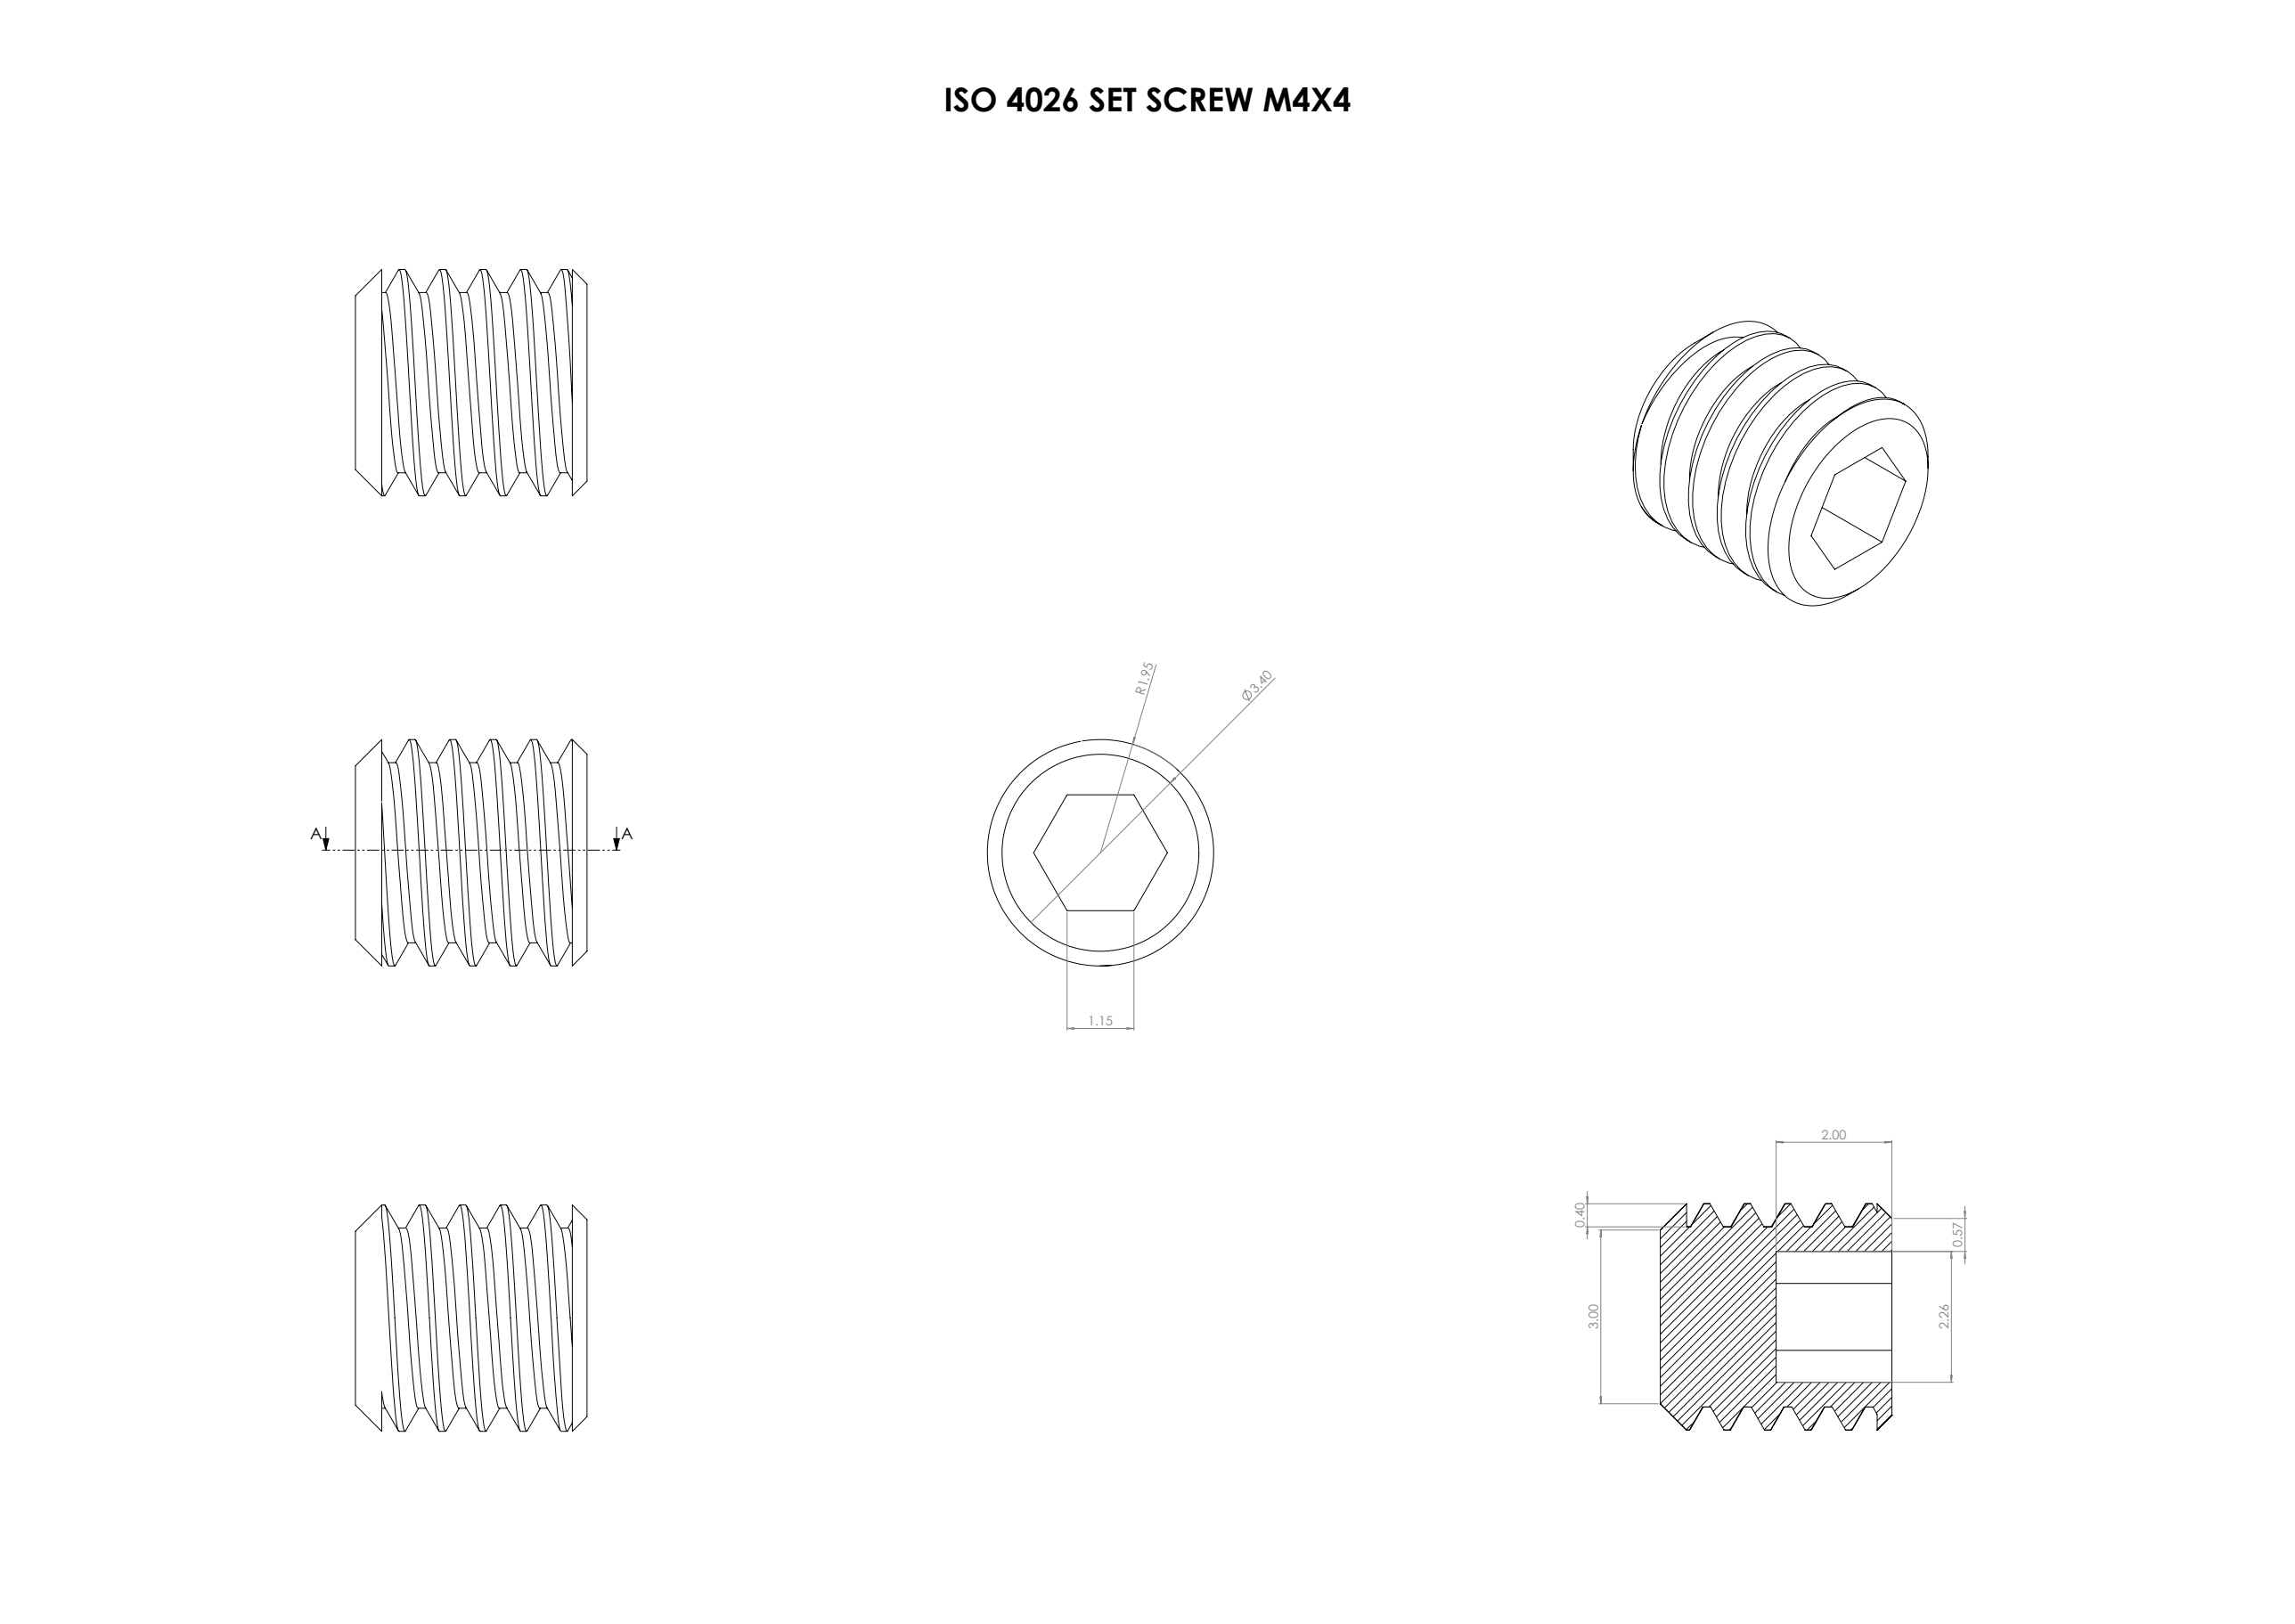
ISO-10303-21;
HEADER;
/* Generated by software containing ST-Developer
 * from STEP Tools, Inc. (www.steptools.com) 
 */

FILE_DESCRIPTION(
/* description */ (''),
/* implementation_level */ '2;1');

FILE_NAME(
/* name */ '10_ISO_4026_Set_Screw_M4x4.step',
/* time_stamp */ '2026-10-21T01:59:45-07:00',
/* author */ (''),
/* organization */ (''),
/* preprocessor_version */ 'ST-DEVELOPER v20.2',
/* originating_system */ 'Autodesk Translation Framework v15.15.0.0',
/* authorisation */ '');

FILE_SCHEMA (('AUTOMOTIVE_DESIGN { 1 0 10303 214 3 1 1 }'));
ENDSEC;

DATA;
#10=MECHANICAL_DESIGN_GEOMETRIC_PRESENTATION_REPRESENTATION('',(#478),#18281);
#184=B_SPLINE_SURFACE_WITH_KNOTS('',3,3,((#15681,#15682,#15683,#15684,#15685,
#15686,#15687,#15688,#15689,#15690,#15691,#15692,#15693,#15694,#15695,#15696,
#15697,#15698,#15699,#15700,#15701,#15702,#15703,#15704,#15705,#15706,#15707,
#15708,#15709,#15710,#15711,#15712,#15713,#15714,#15715),(#15716,#15717,
#15718,#15719,#15720,#15721,#15722,#15723,#15724,#15725,#15726,#15727,#15728,
#15729,#15730,#15731,#15732,#15733,#15734,#15735,#15736,#15737,#15738,#15739,
#15740,#15741,#15742,#15743,#15744,#15745,#15746,#15747,#15748,#15749,#15750),
(#15751,#15752,#15753,#15754,#15755,#15756,#15757,#15758,#15759,#15760,
#15761,#15762,#15763,#15764,#15765,#15766,#15767,#15768,#15769,#15770,#15771,
#15772,#15773,#15774,#15775,#15776,#15777,#15778,#15779,#15780,#15781,#15782,
#15783,#15784,#15785),(#15786,#15787,#15788,#15789,#15790,#15791,#15792,
#15793,#15794,#15795,#15796,#15797,#15798,#15799,#15800,#15801,#15802,#15803,
#15804,#15805,#15806,#15807,#15808,#15809,#15810,#15811,#15812,#15813,#15814,
#15815,#15816,#15817,#15818,#15819,#15820)),.UNSPECIFIED.,.F.,.F.,.F.,(4,
4),(4,1,1,1,1,1,1,1,1,1,1,1,1,1,1,1,1,1,1,1,1,1,1,1,1,1,1,1,1,1,1,1,4),
(0.,0.0460148164544132),(8.31058692273978,9.29852639258487,10.28646586243,
11.274405332275,12.2623448021201,13.2502842719652,14.2382237418103,15.2261632116554,
16.2141026815005,17.2020421513455,18.1899816211906,19.1779210910357,20.1658605608808,
21.1538000307259,22.141739500571,23.129678970416,24.1176184402611,25.1055579101062,
26.0934973799513,27.0814368497964,28.0693763196415,29.0573157894865,30.0452552593316,
31.0331947291767,32.0211341990218,33.0090736688669,33.997013138712,34.9849526085571,
35.9728920784021,36.9608315482472,37.9487710180923,38.9367104879374,39.9246499577825),
 .UNSPECIFIED.);
#185=B_SPLINE_SURFACE_WITH_KNOTS('',3,3,((#16035,#16036,#16037,#16038,#16039,
#16040,#16041,#16042,#16043,#16044,#16045,#16046,#16047,#16048,#16049,#16050,
#16051,#16052,#16053,#16054,#16055,#16056,#16057,#16058,#16059,#16060,#16061,
#16062,#16063,#16064,#16065,#16066,#16067,#16068,#16069),(#16070,#16071,
#16072,#16073,#16074,#16075,#16076,#16077,#16078,#16079,#16080,#16081,#16082,
#16083,#16084,#16085,#16086,#16087,#16088,#16089,#16090,#16091,#16092,#16093,
#16094,#16095,#16096,#16097,#16098,#16099,#16100,#16101,#16102,#16103,#16104),
(#16105,#16106,#16107,#16108,#16109,#16110,#16111,#16112,#16113,#16114,
#16115,#16116,#16117,#16118,#16119,#16120,#16121,#16122,#16123,#16124,#16125,
#16126,#16127,#16128,#16129,#16130,#16131,#16132,#16133,#16134,#16135,#16136,
#16137,#16138,#16139),(#16140,#16141,#16142,#16143,#16144,#16145,#16146,
#16147,#16148,#16149,#16150,#16151,#16152,#16153,#16154,#16155,#16156,#16157,
#16158,#16159,#16160,#16161,#16162,#16163,#16164,#16165,#16166,#16167,#16168,
#16169,#16170,#16171,#16172,#16173,#16174)),.UNSPECIFIED.,.F.,.F.,.F.,(4,
4),(4,1,1,1,1,1,1,1,1,1,1,1,1,1,1,1,1,1,1,1,1,1,1,1,1,1,1,1,1,1,1,1,4),
(0.,0.0460148164544132),(11.6154215191107,12.6033609889557,13.5913004588008,
14.5792399286459,15.567179398491,16.5551188683361,17.5430583381812,18.5309978080262,
19.5189372778713,20.5068767477164,21.4948162175615,22.4827556874066,23.4706951572517,
24.4586346270967,25.4465740969418,26.4345135667869,27.422453036632,28.4103925064771,
29.3983319763222,30.3862714461672,31.3742109160123,32.3621503858574,33.3500898557025,
34.3380293255476,35.3259687953927,36.3139082652377,37.3018477350828,38.2897872049279,
39.277726674773,40.2656661446181,41.2536056144632,42.2415450843083,43.2294845541533),
 .UNSPECIFIED.);
#285=B_SPLINE_CURVE_WITH_KNOTS('',3,(#15173,#15174,#15175,#15176,#15177,
#15178,#15179,#15180,#15181,#15182),.UNSPECIFIED.,.F.,.F.,(4,3,3,4),(-4.09254174883831,
-3.95175787938034,-2.96381840953525,-2.0651401332781),.UNSPECIFIED.);
#286=B_SPLINE_CURVE_WITH_KNOTS('',3,(#15185,#15186,#15187,#15188,#15189,
#15190,#15191),.UNSPECIFIED.,.F.,.F.,(4,3,4),(0.,0.987939469845084,1.11419103802959),
 .UNSPECIFIED.);
#287=B_SPLINE_CURVE_WITH_KNOTS('',3,(#15196,#15197,#15198,#15199,#15200,
#15201,#15202,#15203,#15204,#15205,#15206,#15207,#15208,#15209,#15210,#15211,
#15212,#15213,#15214,#15215,#15216,#15217),.UNSPECIFIED.,.F.,.F.,(4,3,3,
3,3,3,3,4),(-10.3757270560179,-9.87939469845084,-8.89145522860576,-7.90351575876067,
-6.91557628891559,-5.92763681907051,-4.93969734922542,-4.09254174883831),
 .UNSPECIFIED.);
#288=B_SPLINE_CURVE_WITH_KNOTS('',3,(#15218,#15219,#15220,#15221,#15222,
#15223,#15224,#15225,#15226,#15227,#15228,#15229,#15230,#15231,#15232,#15233,
#15234,#15235,#15236,#15237,#15238,#15239),.UNSPECIFIED.,.F.,.F.,(4,3,3,
3,3,3,3,4),(1.11419103802959,1.97587893969017,2.96381840953525,3.95175787938034,
4.93969734922542,5.9276368190705,6.91557628891559,7.39737634520918),
 .UNSPECIFIED.);
#289=B_SPLINE_CURVE_WITH_KNOTS('',3,(#15244,#15245,#15246,#15247,#15248,
#15249,#15250,#15251,#15252,#15253,#15254,#15255,#15256,#15257,#15258,#15259,
#15260,#15261,#15262,#15263,#15264,#15265),.UNSPECIFIED.,.F.,.F.,(4,3,3,
3,3,3,3,4),(-16.6589123631975,-15.8070315175213,-14.8190920476763,-13.8311525778312,
-12.8432131079861,-11.855273638141,-10.8673341682959,-10.3757270560179),
 .UNSPECIFIED.);
#290=B_SPLINE_CURVE_WITH_KNOTS('',3,(#15266,#15267,#15268,#15269,#15270,
#15271,#15272,#15273,#15274,#15275,#15276,#15277,#15278,#15279,#15280,#15281,
#15282,#15283,#15284,#15285,#15286,#15287),.UNSPECIFIED.,.F.,.F.,(4,3,3,
3,3,3,3,4),(7.39737634520918,7.90351575876067,8.89145522860576,9.87939469845084,
10.8673341682959,11.855273638141,12.8432131079861,13.6805616523888),
 .UNSPECIFIED.);
#291=B_SPLINE_CURVE_WITH_KNOTS('',3,(#15292,#15293,#15294,#15295,#15296,
#15297,#15298,#15299,#15300,#15301,#15302,#15303,#15304,#15305,#15306,#15307,
#15308,#15309,#15310,#15311,#15312,#15313,#15314,#15315,#15316),
 .UNSPECIFIED.,.F.,.F.,(4,3,3,3,3,3,3,3,4),(-22.9420976703771,-22.7226078064369,
-21.7346683365918,-20.7467288667468,-19.7587893969017,-18.7708499270566,
-17.7829104572115,-16.7949709873664,-16.6589123631975),.UNSPECIFIED.);
#292=B_SPLINE_CURVE_WITH_KNOTS('',3,(#15317,#15318,#15319,#15320,#15321,
#15322,#15323,#15324,#15325,#15326,#15327,#15328,#15329,#15330,#15331,#15332,
#15333,#15334,#15335,#15336,#15337,#15338,#15339,#15340,#15341),
 .UNSPECIFIED.,.F.,.F.,(4,3,3,3,3,3,3,3,4),(13.6805616523888,13.8311525778312,
14.8190920476763,15.8070315175213,16.7949709873664,17.7829104572115,18.7708499270566,
19.7587893969017,19.9637469595684),.UNSPECIFIED.);
#293=B_SPLINE_CURVE_WITH_KNOTS('',3,(#15346,#15347,#15348,#15349,#15350,
#15351,#15352,#15353,#15354,#15355,#15356,#15357,#15358,#15359,#15360,#15361,
#15362,#15363,#15364,#15365,#15366,#15367),.UNSPECIFIED.,.F.,.F.,(4,3,3,
3,3,3,3,4),(-29.2252829775566,-28.6502446255074,-27.6623051556623,-26.6743656858173,
-25.6864262159722,-24.6984867461271,-23.710547276282,-22.9420976703771),
 .UNSPECIFIED.);
#294=B_SPLINE_CURVE_WITH_KNOTS('',3,(#15368,#15369,#15370,#15371,#15372,
#15373,#15374,#15375,#15376,#15377,#15378,#15379,#15380,#15381,#15382,#15383,
#15384,#15385,#15386,#15387,#15388,#15389),.UNSPECIFIED.,.F.,.F.,(4,3,3,
3,3,3,3,4),(19.9637469595684,20.7467288667468,21.7346683365918,22.7226078064369,
23.710547276282,24.6984867461271,25.6864262159722,26.2469322667479),
 .UNSPECIFIED.);
#295=B_SPLINE_CURVE_WITH_KNOTS('',3,(#15395,#15396,#15397,#15398),
 .UNSPECIFIED.,.F.,.F.,(4,4),(40.8407044966673,41.1643444208752),
 .UNSPECIFIED.);
#296=B_SPLINE_CURVE_WITH_KNOTS('',3,(#15404,#15405,#15406,#15407,#15408,
#15409,#15410,#15411,#15412,#15413),.UNSPECIFIED.,.F.,.F.,(4,1,1,1,1,1,
1,4),(34.5575191894877,35.3259687953927,36.3139082652377,37.3018477350828,
38.2897872049279,39.277726674773,40.2656661446181,40.8407044966673),
 .UNSPECIFIED.);
#297=B_SPLINE_CURVE_WITH_KNOTS('',3,(#15416,#15417,#15418,#15419,#15420,
#15421,#15422,#15423,#15424),.UNSPECIFIED.,.F.,.F.,(4,1,1,1,1,1,4),(34.5575191894877,
34.9849526085571,35.9728920784021,36.9608315482472,37.9487710180923,38.9367104879374,
39.9246499577825),.UNSPECIFIED.);
#298=B_SPLINE_CURVE_WITH_KNOTS('',3,(#15429,#15430,#15431,#15432,#15433,
#15434,#15435,#15436,#15437,#15438,#15439),.UNSPECIFIED.,.F.,.F.,(4,1,1,
1,1,1,1,1,4),(28.2743338823081,28.4103925064771,29.3983319763222,30.3862714461672,
31.3742109160123,32.3621503858574,33.3500898557025,34.3380293255476,34.5575191894877),
 .UNSPECIFIED.);
#299=B_SPLINE_CURVE_WITH_KNOTS('',3,(#15440,#15441,#15442,#15443,#15444,
#15445,#15446,#15447,#15448,#15449),.UNSPECIFIED.,.F.,.F.,(4,1,1,1,1,1,
1,4),(28.2743338823081,29.0573157894865,30.0452552593316,31.0331947291767,
32.0211341990218,33.0090736688669,33.997013138712,34.5575191894877),
 .UNSPECIFIED.);
#300=B_SPLINE_CURVE_WITH_KNOTS('',3,(#15454,#15455,#15456,#15457,#15458,
#15459,#15460,#15461,#15462,#15463),.UNSPECIFIED.,.F.,.F.,(4,1,1,1,1,1,
1,4),(21.9911485751286,22.4827556874066,23.4706951572517,24.4586346270967,
25.4465740969418,26.4345135667869,27.422453036632,28.2743338823081),
 .UNSPECIFIED.);
#301=B_SPLINE_CURVE_WITH_KNOTS('',3,(#15464,#15465,#15466,#15467,#15468,
#15469,#15470,#15471,#15472,#15473,#15474),.UNSPECIFIED.,.F.,.F.,(4,1,1,
1,1,1,1,1,4),(21.9911485751285,22.141739500571,23.129678970416,24.1176184402611,
25.1055579101062,26.0934973799513,27.0814368497964,28.0693763196415,28.2743338823081),
 .UNSPECIFIED.);
#302=B_SPLINE_CURVE_WITH_KNOTS('',3,(#15479,#15480,#15481,#15482,#15483,
#15484,#15485,#15486,#15487,#15488),.UNSPECIFIED.,.F.,.F.,(4,1,1,1,1,1,
1,4),(15.707963267949,16.5551188683361,17.5430583381812,18.5309978080262,
19.5189372778713,20.5068767477164,21.4948162175615,21.9911485751286),
 .UNSPECIFIED.);
#303=B_SPLINE_CURVE_WITH_KNOTS('',3,(#15489,#15490,#15491,#15492,#15493,
#15494,#15495,#15496,#15497,#15498),.UNSPECIFIED.,.F.,.F.,(4,1,1,1,1,1,
1,4),(15.707963267949,16.2141026815005,17.2020421513455,18.1899816211906,
19.1779210910357,20.1658605608808,21.1538000307259,21.9911485751285),
 .UNSPECIFIED.);
#304=B_SPLINE_CURVE_WITH_KNOTS('',3,(#15501,#15502,#15503,#15504,#15505,
#15506,#15507,#15508,#15509,#15510,#15511,#15512,#15513,#15514,#15515,#15516,
#15517,#15518,#15519,#15520,#15521,#15522,#15523,#15524,#15525,#15526,#15527,
#15528,#15529,#15530,#15531,#15532,#15533,#15534,#15535,#15536,#15537,#15538,
#15539,#15540,#15541,#15542,#15543,#15544,#15545,#15546,#15547,#15548,#15549,
#15550,#15551,#15552,#15553,#15554,#15555,#15556,#15557,#15558,#15559,#15560,
#15561,#15562,#15563,#15564,#15565,#15566,#15567,#15568,#15569,#15570,#15571,
#15572,#15573,#15574,#15575,#15576,#15577,#15578,#15579,#15580,#15581,#15582,
#15583,#15584,#15585,#15586,#15587,#15588),.UNSPECIFIED.,.F.,.F.,(4,3,3,
3,3,3,3,3,3,3,3,3,3,3,3,3,3,3,3,3,3,3,3,3,3,3,3,3,3,4),(-0.366397579005854,
-0.352255736410487,-0.334218451541838,-0.328253122886177,-0.324086270819476,
-0.305360245801884,-0.290366742965128,-0.282186410845882,-0.278570970941181,
-0.259174525664227,-0.239360492094141,-0.225873424847565,-0.218279744579071,
-0.21479349407462,-0.194366185320955,-0.185412223107839,-0.1656728542356,
-0.155318300845875,-0.149835977262723,-0.146387185330202,-0.142989257238056,
-0.122499062045188,-0.10158515832526,-0.0805240629991821,-0.0758041242659399,
-0.0722178501685304,-0.050582110738417,-0.0288905415059291,-0.00765380511821571,
0.),.UNSPECIFIED.);
#305=B_SPLINE_CURVE_WITH_KNOTS('',3,(#15593,#15594,#15595,#15596,#15597,
#15598,#15599,#15600,#15601,#15602,#15603,#15604,#15605,#15606,#15607,#15608,
#15609,#15610,#15611,#15612,#15613,#15614,#15615,#15616,#15617,#15618,#15619,
#15620,#15621,#15622,#15623,#15624,#15625,#15626,#15627,#15628,#15629,#15630,
#15631,#15632,#15633,#15634,#15635,#15636,#15637,#15638,#15639,#15640,#15641,
#15642,#15643,#15644,#15645,#15646,#15647,#15648,#15649,#15650,#15651,#15652,
#15653,#15654,#15655,#15656,#15657,#15658,#15659,#15660,#15661,#15662,#15663,
#15664,#15665,#15666,#15667,#15668,#15669,#15670,#15671,#15672,#15673,#15674,
#15675,#15676,#15677,#15678,#15679,#15680),.UNSPECIFIED.,.F.,.F.,(4,3,3,
3,3,3,3,3,3,3,3,3,3,3,3,3,3,3,3,3,3,3,3,3,3,3,3,3,3,4),(-0.364629307890676,
-0.347233186800937,-0.325605321922639,-0.318094543245741,-0.313657346060215,
-0.309559480087559,-0.288242603902967,-0.272777082256873,-0.267225305920237,
-0.263420566366538,-0.24268211184628,-0.222383830675501,-0.20791748069018,
-0.196986121529868,-0.193341724847835,-0.17372888638403,-0.164518430734214,
-0.144479075481155,-0.134892353717832,-0.129096949286913,-0.12579032958573,
-0.106361418226009,-0.0869541719015021,-0.0679077912466892,-0.0628545069907101,
-0.0595313101688987,-0.0409300680615467,-0.0226566529034227,-0.00496781908450919,
0.),.UNSPECIFIED.);
#306=B_SPLINE_CURVE_WITH_KNOTS('',3,(#15821,#15822,#15823,#15824,#15825,
#15826,#15827,#15828,#15829,#15830,#15831,#15832,#15833),.UNSPECIFIED.,
 .F.,.F.,(4,3,3,3,4),(26.2469322667479,26.6743656858173,27.6623051556624,
28.6502446255074,29.5489229017646),.UNSPECIFIED.);
#307=B_SPLINE_CURVE_WITH_KNOTS('',3,(#15835,#15836,#15837,#15838,#15839,
#15840,#15841,#15842,#15843,#15844,#15845,#15846,#15847,#15848,#15849,#15850,
#15851,#15852,#15853,#15854,#15855,#15856,#15857,#15858,#15859,#15860,#15861,
#15862,#15863,#15864,#15865,#15866,#15867,#15868,#15869,#15870,#15871,#15872,
#15873,#15874,#15875,#15876,#15877,#15878,#15879,#15880,#15881,#15882,#15883,
#15884,#15885,#15886,#15887,#15888,#15889,#15890,#15891,#15892,#15893,#15894,
#15895,#15896,#15897,#15898,#15899,#15900,#15901,#15902,#15903,#15904,#15905,
#15906,#15907,#15908,#15909,#15910,#15911,#15912,#15913,#15914,#15915,#15916,
#15917,#15918,#15919,#15920,#15921,#15922),.UNSPECIFIED.,.F.,.F.,(4,3,3,
3,3,3,3,3,3,3,3,3,3,3,3,3,3,3,3,3,3,3,3,3,3,3,3,3,3,4),(-0.366397579005844,
-0.352255736410479,-0.334218432653028,-0.328253038170767,-0.324086234565793,
-0.305360194129425,-0.290366697751727,-0.282186333509408,-0.278570909684785,
-0.259174452080044,-0.239360419305942,-0.225873370256417,-0.218279602851231,
-0.214793320223163,-0.194366011802257,-0.185412223107841,-0.165672847130201,
-0.155318294184563,-0.149835975114951,-0.146387182322352,-0.142989257864255,
-0.122499054249301,-0.101585142121661,-0.0805240463756091,-0.0758040661415852,
-0.0722178274121236,-0.0505820817915926,-0.0288905167825514,-0.00765380478964332,
0.),.UNSPECIFIED.);
#308=B_SPLINE_CURVE_WITH_KNOTS('',3,(#15923,#15924,#15925,#15926,#15927,
#15928,#15929,#15930,#15931),.UNSPECIFIED.,.F.,.F.,(4,1,1,1,1,1,4),(10.3757270560179,
11.274405332275,12.2623448021201,13.2502842719652,14.2382237418103,15.2261632116554,
15.707963267949),.UNSPECIFIED.);
#309=B_SPLINE_CURVE_WITH_KNOTS('',3,(#15937,#15938,#15939,#15940,#15941,
#15942,#15943,#15944,#15945,#15946,#15947,#15948,#15949,#15950,#15951,#15952,
#15953,#15954,#15955,#15956,#15957,#15958,#15959,#15960,#15961,#15962,#15963,
#15964,#15965,#15966,#15967,#15968,#15969,#15970,#15971,#15972,#15973,#15974,
#15975,#15976,#15977,#15978,#15979,#15980,#15981,#15982,#15983,#15984,#15985,
#15986,#15987,#15988,#15989,#15990,#15991,#15992,#15993,#15994,#15995,#15996,
#15997,#15998,#15999,#16000,#16001,#16002,#16003,#16004,#16005,#16006,#16007,
#16008,#16009,#16010,#16011,#16012,#16013,#16014,#16015,#16016,#16017,#16018,
#16019,#16020,#16021,#16022,#16023,#16024),.UNSPECIFIED.,.F.,.F.,(4,3,3,
3,3,3,3,3,3,3,3,3,3,3,3,3,3,3,3,3,3,3,3,3,3,3,3,3,3,4),(-0.364629307890668,
-0.347233186800931,-0.325605321836021,-0.318094550462088,-0.313657357457997,
-0.309559484803747,-0.288242609186508,-0.272777086879971,-0.267225319700862,
-0.263420582037393,-0.242682128922672,-0.222383863217287,-0.207917505096519,
-0.19698615658864,-0.193341780935945,-0.173728958311534,-0.164518430734215,
-0.144479084110425,-0.134892371590082,-0.129097020267292,-0.125790396614882,
-0.106361491905245,-0.0869542352211722,-0.0679078299359471,-0.0628545671260098,
-0.0595313315005194,-0.0409300719336087,-0.0226566308768889,-0.0049677658155539,
0.),.UNSPECIFIED.);
#310=B_SPLINE_CURVE_WITH_KNOTS('',3,(#16027,#16028,#16029,#16030,#16031,
#16032,#16033,#16034),.UNSPECIFIED.,.F.,.F.,(4,1,1,1,1,4),(11.6154215191107,
12.6033609889557,13.5913004588008,14.5792399286459,15.567179398491,15.707963267949),
 .UNSPECIFIED.);
#311=B_SPLINE_CURVE_WITH_KNOTS('',3,(#16175,#16176,#16177,#16178,#16179,
#16180,#16181,#16182,#16183,#16184),.UNSPECIFIED.,.F.,.F.,(4,3,3,4),(-31.6140630350427,
-30.6261235651976,-29.6381840953525,-29.2252829775566),.UNSPECIFIED.);
#430=CONICAL_SURFACE('',#9878,1.75,0.785398163397449);
#431=CONICAL_SURFACE('',#9881,1.85,0.785398163397448);
#447=SHAPE_REPRESENTATION_RELATIONSHIP('SRR','None',#18349,#460);
#460=ADVANCED_BREP_SHAPE_REPRESENTATION('',(#491),#18278);
#478=STYLED_ITEM('',(#18481),#491);
#491=MANIFOLD_SOLID_BREP('Body1',#9095);
#540=CYLINDRICAL_SURFACE('',#9848,1.954);
#541=CYLINDRICAL_SURFACE('',#9850,1.954);
#542=CYLINDRICAL_SURFACE('',#9851,1.954);
#543=CYLINDRICAL_SURFACE('',#9852,1.954);
#544=CYLINDRICAL_SURFACE('',#9853,1.954);
#545=CYLINDRICAL_SURFACE('',#9854,1.5555);
#546=CYLINDRICAL_SURFACE('',#9856,1.5555);
#547=CYLINDRICAL_SURFACE('',#9858,1.5555);
#548=CYLINDRICAL_SURFACE('',#9859,1.5555);
#549=CYLINDRICAL_SURFACE('',#9860,1.5555);
#550=CYLINDRICAL_SURFACE('',#9868,1.5555);
#551=CYLINDRICAL_SURFACE('',#9879,1.954);
#626=FACE_BOUND('',#1886,.T.);
#796=CIRCLE('',#9849,1.954);
#797=CIRCLE('',#9855,1.5555);
#798=CIRCLE('',#9857,1.5555);
#799=CIRCLE('',#9862,1.954);
#800=CIRCLE('',#9863,1.954);
#801=CIRCLE('',#9865,1.954);
#802=CIRCLE('',#9866,1.954);
#803=CIRCLE('',#9867,1.5555);
#804=CIRCLE('',#9877,1.5);
#805=CIRCLE('',#9880,1.954);
#806=CIRCLE('',#9882,1.7);
#1290=FACE_OUTER_BOUND('',#1859,.T.);
#1291=FACE_OUTER_BOUND('',#1860,.T.);
#1292=FACE_OUTER_BOUND('',#1861,.T.);
#1293=FACE_OUTER_BOUND('',#1862,.T.);
#1294=FACE_OUTER_BOUND('',#1863,.T.);
#1295=FACE_OUTER_BOUND('',#1864,.T.);
#1296=FACE_OUTER_BOUND('',#1865,.T.);
#1297=FACE_OUTER_BOUND('',#1866,.T.);
#1298=FACE_OUTER_BOUND('',#1867,.T.);
#1299=FACE_OUTER_BOUND('',#1868,.T.);
#1300=FACE_OUTER_BOUND('',#1869,.T.);
#1301=FACE_OUTER_BOUND('',#1870,.T.);
#1302=FACE_OUTER_BOUND('',#1871,.T.);
#1303=FACE_OUTER_BOUND('',#1872,.T.);
#1304=FACE_OUTER_BOUND('',#1873,.T.);
#1305=FACE_OUTER_BOUND('',#1874,.T.);
#1306=FACE_OUTER_BOUND('',#1875,.T.);
#1307=FACE_OUTER_BOUND('',#1876,.T.);
#1308=FACE_OUTER_BOUND('',#1877,.T.);
#1309=FACE_OUTER_BOUND('',#1878,.T.);
#1310=FACE_OUTER_BOUND('',#1879,.T.);
#1311=FACE_OUTER_BOUND('',#1880,.T.);
#1312=FACE_OUTER_BOUND('',#1881,.T.);
#1313=FACE_OUTER_BOUND('',#1882,.T.);
#1314=FACE_OUTER_BOUND('',#1883,.T.);
#1315=FACE_OUTER_BOUND('',#1884,.T.);
#1316=FACE_OUTER_BOUND('',#1885,.T.);
#1859=EDGE_LOOP('',(#7866,#7867,#7868,#7869));
#1860=EDGE_LOOP('',(#7870,#7871,#7872,#7873));
#1861=EDGE_LOOP('',(#7874,#7875,#7876,#7877));
#1862=EDGE_LOOP('',(#7878,#7879,#7880,#7881));
#1863=EDGE_LOOP('',(#7882,#7883,#7884,#7885));
#1864=EDGE_LOOP('',(#7886,#7887,#7888));
#1865=EDGE_LOOP('',(#7889,#7890,#7891,#7892,#7893));
#1866=EDGE_LOOP('',(#7894,#7895,#7896,#7897));
#1867=EDGE_LOOP('',(#7898,#7899,#7900,#7901));
#1868=EDGE_LOOP('',(#7902,#7903,#7904,#7905));
#1869=EDGE_LOOP('',(#7906,#7907,#7908,#7909,#7910,#7911));
#1870=EDGE_LOOP('',(#7912,#7913,#7914,#7915,#7916,#7917,#7918,#7919,#7920,
#7921,#7922,#7923,#7924));
#1871=EDGE_LOOP('',(#7925,#7926,#7927,#7928,#7929));
#1872=EDGE_LOOP('',(#7930,#7931,#7932,#7933));
#1873=EDGE_LOOP('',(#7934,#7935,#7936,#7937,#7938,#7939,#7940,#7941,#7942,
#7943,#7944,#7945,#7946,#7947));
#1874=EDGE_LOOP('',(#7948,#7949,#7950,#7951));
#1875=EDGE_LOOP('',(#7952,#7953,#7954,#7955));
#1876=EDGE_LOOP('',(#7956,#7957,#7958,#7959));
#1877=EDGE_LOOP('',(#7960,#7961,#7962,#7963));
#1878=EDGE_LOOP('',(#7964,#7965,#7966,#7967));
#1879=EDGE_LOOP('',(#7968,#7969,#7970,#7971));
#1880=EDGE_LOOP('',(#7972,#7973,#7974,#7975,#7976,#7977));
#1881=EDGE_LOOP('',(#7978));
#1882=EDGE_LOOP('',(#7979,#7980,#7981,#7982,#7983,#7984));
#1883=EDGE_LOOP('',(#7985,#7986,#7987,#7988));
#1884=EDGE_LOOP('',(#7989,#7990,#7991,#7992,#7993,#7994));
#1885=EDGE_LOOP('',(#7995));
#1886=EDGE_LOOP('',(#7996,#7997,#7998,#7999,#8000,#8001));
#2703=LINE('',#15171,#3548);
#2704=LINE('',#15195,#3549);
#2705=LINE('',#15243,#3550);
#2706=LINE('',#15291,#3551);
#2707=LINE('',#15345,#3552);
#2708=LINE('',#15393,#3553);
#2709=LINE('',#15403,#3554);
#2710=LINE('',#15428,#3555);
#2711=LINE('',#15453,#3556);
#2712=LINE('',#15478,#3557);
#2713=LINE('',#16188,#3558);
#2714=LINE('',#16190,#3559);
#2715=LINE('',#16192,#3560);
#2716=LINE('',#16193,#3561);
#2717=LINE('',#16196,#3562);
#2718=LINE('',#16198,#3563);
#2719=LINE('',#16199,#3564);
#2720=LINE('',#16202,#3565);
#2721=LINE('',#16204,#3566);
#2722=LINE('',#16205,#3567);
#2723=LINE('',#16208,#3568);
#2724=LINE('',#16210,#3569);
#2725=LINE('',#16211,#3570);
#2726=LINE('',#16214,#3571);
#2727=LINE('',#16216,#3572);
#2728=LINE('',#16217,#3573);
#2729=LINE('',#16219,#3574);
#2730=LINE('',#16220,#3575);
#2731=LINE('',#16226,#3576);
#2732=LINE('',#16232,#3577);
#3548=VECTOR('',#11951,2.);
#3549=VECTOR('',#11956,2.);
#3550=VECTOR('',#11959,2.);
#3551=VECTOR('',#11962,2.);
#3552=VECTOR('',#11965,2.);
#3553=VECTOR('',#11968,1.5555);
#3554=VECTOR('',#11973,1.5555);
#3555=VECTOR('',#11978,1.5555);
#3556=VECTOR('',#11981,1.5555);
#3557=VECTOR('',#11984,1.5555);
#3558=VECTOR('',#12003,10.);
#3559=VECTOR('',#12004,10.);
#3560=VECTOR('',#12005,10.);
#3561=VECTOR('',#12006,10.);
#3562=VECTOR('',#12009,10.);
#3563=VECTOR('',#12010,10.);
#3564=VECTOR('',#12011,10.);
#3565=VECTOR('',#12014,10.);
#3566=VECTOR('',#12015,10.);
#3567=VECTOR('',#12016,10.);
#3568=VECTOR('',#12019,10.);
#3569=VECTOR('',#12020,10.);
#3570=VECTOR('',#12021,10.);
#3571=VECTOR('',#12024,10.);
#3572=VECTOR('',#12025,10.);
#3573=VECTOR('',#12026,10.);
#3574=VECTOR('',#12029,10.);
#3575=VECTOR('',#12030,10.);
#3576=VECTOR('',#12039,1.75);
#3577=VECTOR('',#12048,1.85);
#4296=VERTEX_POINT('',#15169);
#4297=VERTEX_POINT('',#15170);
#4298=VERTEX_POINT('',#15172);
#4299=VERTEX_POINT('',#15183);
#4300=VERTEX_POINT('',#15193);
#4301=VERTEX_POINT('',#15194);
#4302=VERTEX_POINT('',#15241);
#4303=VERTEX_POINT('',#15242);
#4304=VERTEX_POINT('',#15289);
#4305=VERTEX_POINT('',#15290);
#4306=VERTEX_POINT('',#15343);
#4307=VERTEX_POINT('',#15344);
#4308=VERTEX_POINT('',#15391);
#4309=VERTEX_POINT('',#15392);
#4310=VERTEX_POINT('',#15394);
#4311=VERTEX_POINT('',#15401);
#4312=VERTEX_POINT('',#15402);
#4313=VERTEX_POINT('',#15414);
#4314=VERTEX_POINT('',#15426);
#4315=VERTEX_POINT('',#15427);
#4316=VERTEX_POINT('',#15451);
#4317=VERTEX_POINT('',#15452);
#4318=VERTEX_POINT('',#15476);
#4319=VERTEX_POINT('',#15477);
#4320=VERTEX_POINT('',#15500);
#4321=VERTEX_POINT('',#15589);
#4322=VERTEX_POINT('',#15591);
#4323=VERTEX_POINT('',#15834);
#4324=VERTEX_POINT('',#15933);
#4325=VERTEX_POINT('',#15936);
#4326=VERTEX_POINT('',#16186);
#4327=VERTEX_POINT('',#16187);
#4328=VERTEX_POINT('',#16189);
#4329=VERTEX_POINT('',#16191);
#4330=VERTEX_POINT('',#16195);
#4331=VERTEX_POINT('',#16197);
#4332=VERTEX_POINT('',#16201);
#4333=VERTEX_POINT('',#16203);
#4334=VERTEX_POINT('',#16207);
#4335=VERTEX_POINT('',#16209);
#4336=VERTEX_POINT('',#16213);
#4337=VERTEX_POINT('',#16215);
#4338=VERTEX_POINT('',#16223);
#4339=VERTEX_POINT('',#16230);
#5505=EDGE_CURVE('',#4296,#4297,#2703,.T.);
#5506=EDGE_CURVE('',#4296,#4298,#285,.T.);
#5507=EDGE_CURVE('',#4298,#4299,#796,.T.);
#5508=EDGE_CURVE('',#4299,#4297,#286,.T.);
#5509=EDGE_CURVE('',#4300,#4301,#2704,.T.);
#5510=EDGE_CURVE('',#4300,#4296,#287,.T.);
#5511=EDGE_CURVE('',#4297,#4301,#288,.T.);
#5512=EDGE_CURVE('',#4302,#4303,#2705,.T.);
#5513=EDGE_CURVE('',#4302,#4300,#289,.T.);
#5514=EDGE_CURVE('',#4301,#4303,#290,.T.);
#5515=EDGE_CURVE('',#4304,#4305,#2706,.T.);
#5516=EDGE_CURVE('',#4304,#4302,#291,.T.);
#5517=EDGE_CURVE('',#4303,#4305,#292,.T.);
#5518=EDGE_CURVE('',#4306,#4307,#2707,.T.);
#5519=EDGE_CURVE('',#4306,#4304,#293,.T.);
#5520=EDGE_CURVE('',#4305,#4307,#294,.T.);
#5521=EDGE_CURVE('',#4308,#4309,#2708,.T.);
#5522=EDGE_CURVE('',#4308,#4310,#295,.T.);
#5523=EDGE_CURVE('',#4309,#4310,#797,.T.);
#5524=EDGE_CURVE('',#4311,#4312,#2709,.T.);
#5525=EDGE_CURVE('',#4311,#4308,#296,.T.);
#5526=EDGE_CURVE('',#4313,#4309,#798,.T.);
#5527=EDGE_CURVE('',#4312,#4313,#297,.T.);
#5528=EDGE_CURVE('',#4314,#4315,#2710,.T.);
#5529=EDGE_CURVE('',#4314,#4311,#298,.T.);
#5530=EDGE_CURVE('',#4315,#4312,#299,.T.);
#5531=EDGE_CURVE('',#4316,#4317,#2711,.T.);
#5532=EDGE_CURVE('',#4316,#4314,#300,.T.);
#5533=EDGE_CURVE('',#4317,#4315,#301,.T.);
#5534=EDGE_CURVE('',#4318,#4319,#2712,.T.);
#5535=EDGE_CURVE('',#4318,#4316,#302,.T.);
#5536=EDGE_CURVE('',#4319,#4317,#303,.T.);
#5537=EDGE_CURVE('',#4310,#4320,#304,.T.);
#5538=EDGE_CURVE('',#4321,#4320,#799,.F.);
#5539=EDGE_CURVE('',#4322,#4321,#800,.F.);
#5540=EDGE_CURVE('',#4322,#4313,#305,.T.);
#5541=EDGE_CURVE('',#4307,#4322,#306,.T.);
#5542=EDGE_CURVE('',#4323,#4299,#307,.T.);
#5543=EDGE_CURVE('',#4323,#4319,#308,.T.);
#5544=EDGE_CURVE('',#4299,#4324,#801,.T.);
#5545=EDGE_CURVE('',#4324,#4298,#802,.T.);
#5546=EDGE_CURVE('',#4298,#4325,#309,.T.);
#5547=EDGE_CURVE('',#4325,#4323,#803,.T.);
#5548=EDGE_CURVE('',#4325,#4318,#310,.T.);
#5549=EDGE_CURVE('',#4320,#4306,#311,.T.);
#5550=EDGE_CURVE('',#4326,#4327,#2713,.T.);
#5551=EDGE_CURVE('',#4326,#4328,#2714,.T.);
#5552=EDGE_CURVE('',#4328,#4329,#2715,.T.);
#5553=EDGE_CURVE('',#4327,#4329,#2716,.T.);
#5554=EDGE_CURVE('',#4330,#4326,#2717,.T.);
#5555=EDGE_CURVE('',#4330,#4331,#2718,.T.);
#5556=EDGE_CURVE('',#4331,#4328,#2719,.T.);
#5557=EDGE_CURVE('',#4332,#4330,#2720,.T.);
#5558=EDGE_CURVE('',#4332,#4333,#2721,.T.);
#5559=EDGE_CURVE('',#4333,#4331,#2722,.T.);
#5560=EDGE_CURVE('',#4334,#4332,#2723,.T.);
#5561=EDGE_CURVE('',#4334,#4335,#2724,.T.);
#5562=EDGE_CURVE('',#4335,#4333,#2725,.T.);
#5563=EDGE_CURVE('',#4336,#4334,#2726,.T.);
#5564=EDGE_CURVE('',#4336,#4337,#2727,.T.);
#5565=EDGE_CURVE('',#4337,#4335,#2728,.T.);
#5566=EDGE_CURVE('',#4327,#4336,#2729,.T.);
#5567=EDGE_CURVE('',#4329,#4337,#2730,.T.);
#5568=EDGE_CURVE('',#4338,#4338,#804,.T.);
#5569=EDGE_CURVE('',#4324,#4338,#2731,.T.);
#5570=EDGE_CURVE('',#4320,#4322,#805,.F.);
#5571=EDGE_CURVE('',#4339,#4339,#806,.T.);
#5572=EDGE_CURVE('',#4339,#4321,#2732,.T.);
#7866=ORIENTED_EDGE('',*,*,#5505,.F.);
#7867=ORIENTED_EDGE('',*,*,#5506,.T.);
#7868=ORIENTED_EDGE('',*,*,#5507,.T.);
#7869=ORIENTED_EDGE('',*,*,#5508,.T.);
#7870=ORIENTED_EDGE('',*,*,#5509,.F.);
#7871=ORIENTED_EDGE('',*,*,#5510,.T.);
#7872=ORIENTED_EDGE('',*,*,#5505,.T.);
#7873=ORIENTED_EDGE('',*,*,#5511,.T.);
#7874=ORIENTED_EDGE('',*,*,#5512,.F.);
#7875=ORIENTED_EDGE('',*,*,#5513,.T.);
#7876=ORIENTED_EDGE('',*,*,#5509,.T.);
#7877=ORIENTED_EDGE('',*,*,#5514,.T.);
#7878=ORIENTED_EDGE('',*,*,#5515,.F.);
#7879=ORIENTED_EDGE('',*,*,#5516,.T.);
#7880=ORIENTED_EDGE('',*,*,#5512,.T.);
#7881=ORIENTED_EDGE('',*,*,#5517,.T.);
#7882=ORIENTED_EDGE('',*,*,#5518,.F.);
#7883=ORIENTED_EDGE('',*,*,#5519,.T.);
#7884=ORIENTED_EDGE('',*,*,#5515,.T.);
#7885=ORIENTED_EDGE('',*,*,#5520,.T.);
#7886=ORIENTED_EDGE('',*,*,#5521,.F.);
#7887=ORIENTED_EDGE('',*,*,#5522,.T.);
#7888=ORIENTED_EDGE('',*,*,#5523,.F.);
#7889=ORIENTED_EDGE('',*,*,#5524,.F.);
#7890=ORIENTED_EDGE('',*,*,#5525,.T.);
#7891=ORIENTED_EDGE('',*,*,#5521,.T.);
#7892=ORIENTED_EDGE('',*,*,#5526,.F.);
#7893=ORIENTED_EDGE('',*,*,#5527,.F.);
#7894=ORIENTED_EDGE('',*,*,#5528,.F.);
#7895=ORIENTED_EDGE('',*,*,#5529,.T.);
#7896=ORIENTED_EDGE('',*,*,#5524,.T.);
#7897=ORIENTED_EDGE('',*,*,#5530,.F.);
#7898=ORIENTED_EDGE('',*,*,#5531,.F.);
#7899=ORIENTED_EDGE('',*,*,#5532,.T.);
#7900=ORIENTED_EDGE('',*,*,#5528,.T.);
#7901=ORIENTED_EDGE('',*,*,#5533,.F.);
#7902=ORIENTED_EDGE('',*,*,#5534,.F.);
#7903=ORIENTED_EDGE('',*,*,#5535,.T.);
#7904=ORIENTED_EDGE('',*,*,#5531,.T.);
#7905=ORIENTED_EDGE('',*,*,#5536,.F.);
#7906=ORIENTED_EDGE('',*,*,#5526,.T.);
#7907=ORIENTED_EDGE('',*,*,#5523,.T.);
#7908=ORIENTED_EDGE('',*,*,#5537,.T.);
#7909=ORIENTED_EDGE('',*,*,#5538,.F.);
#7910=ORIENTED_EDGE('',*,*,#5539,.F.);
#7911=ORIENTED_EDGE('',*,*,#5540,.T.);
#7912=ORIENTED_EDGE('',*,*,#5540,.F.);
#7913=ORIENTED_EDGE('',*,*,#5541,.F.);
#7914=ORIENTED_EDGE('',*,*,#5520,.F.);
#7915=ORIENTED_EDGE('',*,*,#5517,.F.);
#7916=ORIENTED_EDGE('',*,*,#5514,.F.);
#7917=ORIENTED_EDGE('',*,*,#5511,.F.);
#7918=ORIENTED_EDGE('',*,*,#5508,.F.);
#7919=ORIENTED_EDGE('',*,*,#5542,.F.);
#7920=ORIENTED_EDGE('',*,*,#5543,.T.);
#7921=ORIENTED_EDGE('',*,*,#5536,.T.);
#7922=ORIENTED_EDGE('',*,*,#5533,.T.);
#7923=ORIENTED_EDGE('',*,*,#5530,.T.);
#7924=ORIENTED_EDGE('',*,*,#5527,.T.);
#7925=ORIENTED_EDGE('',*,*,#5544,.T.);
#7926=ORIENTED_EDGE('',*,*,#5545,.T.);
#7927=ORIENTED_EDGE('',*,*,#5546,.T.);
#7928=ORIENTED_EDGE('',*,*,#5547,.T.);
#7929=ORIENTED_EDGE('',*,*,#5542,.T.);
#7930=ORIENTED_EDGE('',*,*,#5534,.T.);
#7931=ORIENTED_EDGE('',*,*,#5543,.F.);
#7932=ORIENTED_EDGE('',*,*,#5547,.F.);
#7933=ORIENTED_EDGE('',*,*,#5548,.T.);
#7934=ORIENTED_EDGE('',*,*,#5537,.F.);
#7935=ORIENTED_EDGE('',*,*,#5522,.F.);
#7936=ORIENTED_EDGE('',*,*,#5525,.F.);
#7937=ORIENTED_EDGE('',*,*,#5529,.F.);
#7938=ORIENTED_EDGE('',*,*,#5532,.F.);
#7939=ORIENTED_EDGE('',*,*,#5535,.F.);
#7940=ORIENTED_EDGE('',*,*,#5548,.F.);
#7941=ORIENTED_EDGE('',*,*,#5546,.F.);
#7942=ORIENTED_EDGE('',*,*,#5506,.F.);
#7943=ORIENTED_EDGE('',*,*,#5510,.F.);
#7944=ORIENTED_EDGE('',*,*,#5513,.F.);
#7945=ORIENTED_EDGE('',*,*,#5516,.F.);
#7946=ORIENTED_EDGE('',*,*,#5519,.F.);
#7947=ORIENTED_EDGE('',*,*,#5549,.F.);
#7948=ORIENTED_EDGE('',*,*,#5550,.F.);
#7949=ORIENTED_EDGE('',*,*,#5551,.T.);
#7950=ORIENTED_EDGE('',*,*,#5552,.T.);
#7951=ORIENTED_EDGE('',*,*,#5553,.F.);
#7952=ORIENTED_EDGE('',*,*,#5554,.F.);
#7953=ORIENTED_EDGE('',*,*,#5555,.T.);
#7954=ORIENTED_EDGE('',*,*,#5556,.T.);
#7955=ORIENTED_EDGE('',*,*,#5551,.F.);
#7956=ORIENTED_EDGE('',*,*,#5557,.F.);
#7957=ORIENTED_EDGE('',*,*,#5558,.T.);
#7958=ORIENTED_EDGE('',*,*,#5559,.T.);
#7959=ORIENTED_EDGE('',*,*,#5555,.F.);
#7960=ORIENTED_EDGE('',*,*,#5560,.F.);
#7961=ORIENTED_EDGE('',*,*,#5561,.T.);
#7962=ORIENTED_EDGE('',*,*,#5562,.T.);
#7963=ORIENTED_EDGE('',*,*,#5558,.F.);
#7964=ORIENTED_EDGE('',*,*,#5563,.F.);
#7965=ORIENTED_EDGE('',*,*,#5564,.T.);
#7966=ORIENTED_EDGE('',*,*,#5565,.T.);
#7967=ORIENTED_EDGE('',*,*,#5561,.F.);
#7968=ORIENTED_EDGE('',*,*,#5566,.F.);
#7969=ORIENTED_EDGE('',*,*,#5553,.T.);
#7970=ORIENTED_EDGE('',*,*,#5567,.T.);
#7971=ORIENTED_EDGE('',*,*,#5564,.F.);
#7972=ORIENTED_EDGE('',*,*,#5567,.F.);
#7973=ORIENTED_EDGE('',*,*,#5552,.F.);
#7974=ORIENTED_EDGE('',*,*,#5556,.F.);
#7975=ORIENTED_EDGE('',*,*,#5559,.F.);
#7976=ORIENTED_EDGE('',*,*,#5562,.F.);
#7977=ORIENTED_EDGE('',*,*,#5565,.F.);
#7978=ORIENTED_EDGE('',*,*,#5568,.F.);
#7979=ORIENTED_EDGE('',*,*,#5544,.F.);
#7980=ORIENTED_EDGE('',*,*,#5507,.F.);
#7981=ORIENTED_EDGE('',*,*,#5545,.F.);
#7982=ORIENTED_EDGE('',*,*,#5569,.T.);
#7983=ORIENTED_EDGE('',*,*,#5568,.T.);
#7984=ORIENTED_EDGE('',*,*,#5569,.F.);
#7985=ORIENTED_EDGE('',*,*,#5518,.T.);
#7986=ORIENTED_EDGE('',*,*,#5541,.T.);
#7987=ORIENTED_EDGE('',*,*,#5570,.F.);
#7988=ORIENTED_EDGE('',*,*,#5549,.T.);
#7989=ORIENTED_EDGE('',*,*,#5571,.F.);
#7990=ORIENTED_EDGE('',*,*,#5572,.T.);
#7991=ORIENTED_EDGE('',*,*,#5538,.T.);
#7992=ORIENTED_EDGE('',*,*,#5570,.T.);
#7993=ORIENTED_EDGE('',*,*,#5539,.T.);
#7994=ORIENTED_EDGE('',*,*,#5572,.F.);
#7995=ORIENTED_EDGE('',*,*,#5571,.T.);
#7996=ORIENTED_EDGE('',*,*,#5550,.T.);
#7997=ORIENTED_EDGE('',*,*,#5566,.T.);
#7998=ORIENTED_EDGE('',*,*,#5563,.T.);
#7999=ORIENTED_EDGE('',*,*,#5560,.T.);
#8000=ORIENTED_EDGE('',*,*,#5557,.T.);
#8001=ORIENTED_EDGE('',*,*,#5554,.T.);
#8539=PLANE('',#9861);
#8540=PLANE('',#9864);
#8541=PLANE('',#9869);
#8542=PLANE('',#9870);
#8543=PLANE('',#9871);
#8544=PLANE('',#9872);
#8545=PLANE('',#9873);
#8546=PLANE('',#9874);
#8547=PLANE('',#9875);
#8548=PLANE('',#9876);
#8549=PLANE('',#9883);
#9011=ADVANCED_FACE('',(#1290),#540,.T.);
#9012=ADVANCED_FACE('',(#1291),#541,.T.);
#9013=ADVANCED_FACE('',(#1292),#542,.T.);
#9014=ADVANCED_FACE('',(#1293),#543,.T.);
#9015=ADVANCED_FACE('',(#1294),#544,.T.);
#9016=ADVANCED_FACE('',(#1295),#545,.T.);
#9017=ADVANCED_FACE('',(#1296),#546,.T.);
#9018=ADVANCED_FACE('',(#1297),#547,.T.);
#9019=ADVANCED_FACE('',(#1298),#548,.T.);
#9020=ADVANCED_FACE('',(#1299),#549,.T.);
#9021=ADVANCED_FACE('',(#1300),#8539,.F.);
#9022=ADVANCED_FACE('',(#1301),#184,.F.);
#9023=ADVANCED_FACE('',(#1302),#8540,.T.);
#9024=ADVANCED_FACE('',(#1303),#550,.T.);
#9025=ADVANCED_FACE('',(#1304),#185,.F.);
#9026=ADVANCED_FACE('',(#1305),#8541,.F.);
#9027=ADVANCED_FACE('',(#1306),#8542,.F.);
#9028=ADVANCED_FACE('',(#1307),#8543,.F.);
#9029=ADVANCED_FACE('',(#1308),#8544,.F.);
#9030=ADVANCED_FACE('',(#1309),#8545,.F.);
#9031=ADVANCED_FACE('',(#1310),#8546,.F.);
#9032=ADVANCED_FACE('',(#1311),#8547,.F.);
#9033=ADVANCED_FACE('',(#1312),#8548,.T.);
#9034=ADVANCED_FACE('',(#1313),#430,.T.);
#9035=ADVANCED_FACE('',(#1314),#551,.T.);
#9036=ADVANCED_FACE('',(#1315),#431,.T.);
#9037=ADVANCED_FACE('',(#1316,#626),#8549,.T.);
#9095=CLOSED_SHELL('',(#9011,#9012,#9013,#9014,#9015,#9016,#9017,#9018,
#9019,#9020,#9021,#9022,#9023,#9024,#9025,#9026,#9027,#9028,#9029,#9030,
#9031,#9032,#9033,#9034,#9035,#9036,#9037));
#9847=AXIS2_PLACEMENT_3D('',#15167,#11947,#11948);
#9848=AXIS2_PLACEMENT_3D('',#15168,#11949,#11950);
#9849=AXIS2_PLACEMENT_3D('',#15184,#11952,#11953);
#9850=AXIS2_PLACEMENT_3D('',#15192,#11954,#11955);
#9851=AXIS2_PLACEMENT_3D('',#15240,#11957,#11958);
#9852=AXIS2_PLACEMENT_3D('',#15288,#11960,#11961);
#9853=AXIS2_PLACEMENT_3D('',#15342,#11963,#11964);
#9854=AXIS2_PLACEMENT_3D('',#15390,#11966,#11967);
#9855=AXIS2_PLACEMENT_3D('',#15399,#11969,#11970);
#9856=AXIS2_PLACEMENT_3D('',#15400,#11971,#11972);
#9857=AXIS2_PLACEMENT_3D('',#15415,#11974,#11975);
#9858=AXIS2_PLACEMENT_3D('',#15425,#11976,#11977);
#9859=AXIS2_PLACEMENT_3D('',#15450,#11979,#11980);
#9860=AXIS2_PLACEMENT_3D('',#15475,#11982,#11983);
#9861=AXIS2_PLACEMENT_3D('',#15499,#11985,#11986);
#9862=AXIS2_PLACEMENT_3D('',#15590,#11987,#11988);
#9863=AXIS2_PLACEMENT_3D('',#15592,#11989,#11990);
#9864=AXIS2_PLACEMENT_3D('',#15932,#11991,#11992);
#9865=AXIS2_PLACEMENT_3D('',#15934,#11993,#11994);
#9866=AXIS2_PLACEMENT_3D('',#15935,#11995,#11996);
#9867=AXIS2_PLACEMENT_3D('',#16025,#11997,#11998);
#9868=AXIS2_PLACEMENT_3D('',#16026,#11999,#12000);
#9869=AXIS2_PLACEMENT_3D('',#16185,#12001,#12002);
#9870=AXIS2_PLACEMENT_3D('',#16194,#12007,#12008);
#9871=AXIS2_PLACEMENT_3D('',#16200,#12012,#12013);
#9872=AXIS2_PLACEMENT_3D('',#16206,#12017,#12018);
#9873=AXIS2_PLACEMENT_3D('',#16212,#12022,#12023);
#9874=AXIS2_PLACEMENT_3D('',#16218,#12027,#12028);
#9875=AXIS2_PLACEMENT_3D('',#16221,#12031,#12032);
#9876=AXIS2_PLACEMENT_3D('',#16222,#12033,#12034);
#9877=AXIS2_PLACEMENT_3D('',#16224,#12035,#12036);
#9878=AXIS2_PLACEMENT_3D('',#16225,#12037,#12038);
#9879=AXIS2_PLACEMENT_3D('',#16227,#12040,#12041);
#9880=AXIS2_PLACEMENT_3D('',#16228,#12042,#12043);
#9881=AXIS2_PLACEMENT_3D('',#16229,#12044,#12045);
#9882=AXIS2_PLACEMENT_3D('',#16231,#12046,#12047);
#9883=AXIS2_PLACEMENT_3D('',#16233,#12049,#12050);
#11947=DIRECTION('axis',(0.,0.,1.));
#11948=DIRECTION('refdir',(1.,0.,0.));
#11949=DIRECTION('center_axis',(1.,0.,0.));
#11950=DIRECTION('ref_axis',(0.,1.,0.));
#11951=DIRECTION('',(-1.,0.,0.));
#11952=DIRECTION('center_axis',(1.,0.,0.));
#11953=DIRECTION('ref_axis',(0.,1.,0.));
#11954=DIRECTION('center_axis',(1.,0.,0.));
#11955=DIRECTION('ref_axis',(0.,1.,0.));
#11956=DIRECTION('',(-1.,0.,0.));
#11957=DIRECTION('center_axis',(1.,0.,0.));
#11958=DIRECTION('ref_axis',(0.,1.,0.));
#11959=DIRECTION('',(-1.,0.,0.));
#11960=DIRECTION('center_axis',(1.,0.,0.));
#11961=DIRECTION('ref_axis',(0.,1.,0.));
#11962=DIRECTION('',(-1.,0.,0.));
#11963=DIRECTION('center_axis',(1.,0.,0.));
#11964=DIRECTION('ref_axis',(0.,1.,0.));
#11965=DIRECTION('',(-1.,0.,0.));
#11966=DIRECTION('center_axis',(1.,0.,0.));
#11967=DIRECTION('ref_axis',(0.,1.,4.77055255383026E-15));
#11968=DIRECTION('',(1.,0.,0.));
#11969=DIRECTION('center_axis',(1.,0.,0.));
#11970=DIRECTION('ref_axis',(0.,1.,4.77055255383026E-15));
#11971=DIRECTION('center_axis',(1.,0.,0.));
#11972=DIRECTION('ref_axis',(0.,1.,4.77055255383026E-15));
#11973=DIRECTION('',(1.,0.,0.));
#11974=DIRECTION('center_axis',(1.,0.,0.));
#11975=DIRECTION('ref_axis',(0.,1.,4.77055255383026E-15));
#11976=DIRECTION('center_axis',(1.,0.,0.));
#11977=DIRECTION('ref_axis',(0.,1.,4.77055255383026E-15));
#11978=DIRECTION('',(1.,0.,0.));
#11979=DIRECTION('center_axis',(1.,0.,0.));
#11980=DIRECTION('ref_axis',(0.,1.,4.77055255383026E-15));
#11981=DIRECTION('',(1.,0.,0.));
#11982=DIRECTION('center_axis',(1.,0.,0.));
#11983=DIRECTION('ref_axis',(0.,1.,4.77055255383026E-15));
#11984=DIRECTION('',(1.,0.,0.));
#11985=DIRECTION('center_axis',(1.,0.,0.));
#11986=DIRECTION('ref_axis',(0.,0.,-1.));
#11987=DIRECTION('center_axis',(-1.,0.,0.));
#11988=DIRECTION('ref_axis',(0.,1.,0.));
#11989=DIRECTION('center_axis',(-1.,0.,0.));
#11990=DIRECTION('ref_axis',(0.,1.,0.));
#11991=DIRECTION('center_axis',(1.,0.,0.));
#11992=DIRECTION('ref_axis',(0.,0.,-1.));
#11993=DIRECTION('center_axis',(1.,0.,0.));
#11994=DIRECTION('ref_axis',(0.,1.,0.));
#11995=DIRECTION('center_axis',(1.,0.,0.));
#11996=DIRECTION('ref_axis',(0.,1.,0.));
#11997=DIRECTION('center_axis',(-1.,0.,0.));
#11998=DIRECTION('ref_axis',(0.,1.,4.77055255383026E-15));
#11999=DIRECTION('center_axis',(1.,0.,0.));
#12000=DIRECTION('ref_axis',(0.,1.,4.77055255383026E-15));
#12001=DIRECTION('center_axis',(0.,0.5,0.866025403784439));
#12002=DIRECTION('ref_axis',(0.,0.866025403784439,-0.5));
#12003=DIRECTION('',(0.,0.866025403784439,-0.5));
#12004=DIRECTION('',(-1.,0.,0.));
#12005=DIRECTION('',(0.,0.866025403784439,-0.5));
#12006=DIRECTION('',(-1.,0.,0.));
#12007=DIRECTION('center_axis',(0.,-0.5,0.866025403784439));
#12008=DIRECTION('ref_axis',(0.,0.866025403784439,0.5));
#12009=DIRECTION('',(0.,0.866025403784439,0.5));
#12010=DIRECTION('',(-1.,0.,0.));
#12011=DIRECTION('',(0.,0.866025403784439,0.5));
#12012=DIRECTION('center_axis',(0.,-1.,-1.20185167898973E-16));
#12013=DIRECTION('ref_axis',(0.,-1.20185167898973E-16,1.));
#12014=DIRECTION('',(0.,-1.20185167898973E-16,1.));
#12015=DIRECTION('',(-1.,0.,0.));
#12016=DIRECTION('',(0.,-1.20185167898973E-16,1.));
#12017=DIRECTION('center_axis',(0.,-0.5,-0.866025403784439));
#12018=DIRECTION('ref_axis',(0.,-0.866025403784439,0.5));
#12019=DIRECTION('',(0.,-0.866025403784439,0.5));
#12020=DIRECTION('',(-1.,0.,0.));
#12021=DIRECTION('',(0.,-0.866025403784439,0.5));
#12022=DIRECTION('center_axis',(0.,0.5,-0.866025403784439));
#12023=DIRECTION('ref_axis',(0.,-0.866025403784439,-0.5));
#12024=DIRECTION('',(0.,-0.866025403784439,-0.5));
#12025=DIRECTION('',(-1.,0.,0.));
#12026=DIRECTION('',(0.,-0.866025403784439,-0.5));
#12027=DIRECTION('center_axis',(0.,1.,-3.60555503696918E-16));
#12028=DIRECTION('ref_axis',(0.,-3.60555503696918E-16,-1.));
#12029=DIRECTION('',(0.,-3.60555503696918E-16,-1.));
#12030=DIRECTION('',(0.,-3.60555503696918E-16,-1.));
#12031=DIRECTION('center_axis',(-1.,0.,0.));
#12032=DIRECTION('ref_axis',(0.,0.,1.));
#12033=DIRECTION('center_axis',(-1.,0.,0.));
#12034=DIRECTION('ref_axis',(0.,0.,1.));
#12035=DIRECTION('center_axis',(1.,0.,0.));
#12036=DIRECTION('ref_axis',(0.,0.,-1.));
#12037=DIRECTION('center_axis',(1.,0.,0.));
#12038=DIRECTION('ref_axis',(0.,1.,0.));
#12039=DIRECTION('',(-0.707106781186547,0.707106781186548,8.65956056235494E-17));
#12040=DIRECTION('center_axis',(1.,0.,0.));
#12041=DIRECTION('ref_axis',(0.,1.,0.));
#12042=DIRECTION('center_axis',(-1.,0.,0.));
#12043=DIRECTION('ref_axis',(0.,1.,0.));
#12044=DIRECTION('center_axis',(-1.,0.,0.));
#12045=DIRECTION('ref_axis',(0.,1.,0.));
#12046=DIRECTION('center_axis',(1.,0.,0.));
#12047=DIRECTION('ref_axis',(0.,0.,-1.));
#12048=DIRECTION('',(-0.707106781186548,-0.707106781186548,-8.65956056235493E-17));
#12049=DIRECTION('center_axis',(1.,0.,0.));
#12050=DIRECTION('ref_axis',(0.,0.,-1.));
#15167=CARTESIAN_POINT('',(0.,0.,0.));
#15168=CARTESIAN_POINT('Origin',(2.1,0.,0.));
#15169=CARTESIAN_POINT('',(0.67986969212423,-1.9556340392028,0.00150612460811491));
#15170=CARTESIAN_POINT('',(0.57813030787577,-1.95561149193597,0.00205040622396644));
#15171=CARTESIAN_POINT('',(2.1,-1.954,-2.39295984553393E-16));
#15172=CARTESIAN_POINT('',(0.454,0.862538756400936,1.75492334225908));
#15173=CARTESIAN_POINT('Ctrl Pts',(0.67986969212423,-1.9556340392028,0.00150612460811491));
#15174=CARTESIAN_POINT('Ctrl Pts',(0.674641520753467,-1.95636945939027,
0.0929737669686619));
#15175=CARTESIAN_POINT('Ctrl Pts',(0.669413349382705,-1.95049672599127,
0.184341808759358));
#15176=CARTESIAN_POINT('Ctrl Pts',(0.664185178011942,-1.937688635782,0.274720676660528));
#15177=CARTESIAN_POINT('Ctrl Pts',(0.627496906321608,-1.84780889387837,
0.908947106032384));
#15178=CARTESIAN_POINT('Ctrl Pts',(0.590808634631275,-1.41640321821628,
1.49446248195575));
#15179=CARTESIAN_POINT('Ctrl Pts',(0.554120362940941,-0.837299495544021,
1.76873092177168));
#15180=CARTESIAN_POINT('Ctrl Pts',(0.520746908627294,-0.310518299782289,
2.01821896860936));
#15181=CARTESIAN_POINT('Ctrl Pts',(0.487373454313647,0.33847734856006,2.01016214817372));
#15182=CARTESIAN_POINT('Ctrl Pts',(0.454,0.863551653131349,1.75602537289061));
#15183=CARTESIAN_POINT('',(0.454,-0.861525859670523,1.75382131162755));
#15184=CARTESIAN_POINT('Origin',(0.454000000000001,0.,0.));
#15185=CARTESIAN_POINT('Ctrl Pts',(0.454,-0.861525859670525,1.75382131162755));
#15186=CARTESIAN_POINT('Ctrl Pts',(0.490688271690334,-1.4390822919413,1.47010951127397));
#15187=CARTESIAN_POINT('Ctrl Pts',(0.527376543380669,-1.86090523699116,
0.881484043774334));
#15188=CARTESIAN_POINT('Ctrl Pts',(0.564064815071003,-1.94128220444048,
0.246930232721736));
#15189=CARTESIAN_POINT('Ctrl Pts',(0.568753312672592,-1.95155380355776,
0.165838813471721));
#15190=CARTESIAN_POINT('Ctrl Pts',(0.573441810274181,-1.95624924699569,
0.0839973382522469));
#15191=CARTESIAN_POINT('Ctrl Pts',(0.57813030787577,-1.95561149193597,0.00205040622396644));
#15192=CARTESIAN_POINT('Origin',(2.1,0.,0.));
#15193=CARTESIAN_POINT('',(1.37986969212423,-1.95093233439697,-2.27181786092989E-5));
#15194=CARTESIAN_POINT('',(1.27813030787577,-1.95093620579234,0.000136491009683568));
#15195=CARTESIAN_POINT('',(2.1,-1.954,-2.39295984553393E-16));
#15196=CARTESIAN_POINT('Ctrl Pts',(1.37986969212423,-1.95093233439697,-2.27181786092989E-5));
#15197=CARTESIAN_POINT('Ctrl Pts',(1.36143781756214,-1.95089544086302,0.324452095312547));
#15198=CARTESIAN_POINT('Ctrl Pts',(1.34300594300005,-1.8741920465679,0.648942870541793));
#15199=CARTESIAN_POINT('Ctrl Pts',(1.32457406843796,-1.72092037455472,0.931966401256464));
#15200=CARTESIAN_POINT('Ctrl Pts',(1.28788579674762,-1.41583622663974,1.49531898672669));
#15201=CARTESIAN_POINT('Ctrl Pts',(1.25119752505729,-0.807387847480595,
1.89437796224664));
#15202=CARTESIAN_POINT('Ctrl Pts',(1.21450925336695,-0.169124111500478,
1.94974527786031));
#15203=CARTESIAN_POINT('Ctrl Pts',(1.17782098167662,0.469139624479642,2.00511259347399));
#15204=CARTESIAN_POINT('Ctrl Pts',(1.14113270998628,1.13721871728073,1.71678824918138));
#15205=CARTESIAN_POINT('Ctrl Pts',(1.10444443829595,1.53474739736028,1.21437219896546));
#15206=CARTESIAN_POINT('Ctrl Pts',(1.06775616660562,1.93227607743982,0.711956148749533));
#15207=CARTESIAN_POINT('Ctrl Pts',(1.03106789491528,2.05925434479783,-0.00455160738971262));
#15208=CARTESIAN_POINT('Ctrl Pts',(0.994379623224949,1.85860375663964,-0.612964951193619));
#15209=CARTESIAN_POINT('Ctrl Pts',(0.957691351534615,1.65795316848146,-1.22137829499753));
#15210=CARTESIAN_POINT('Ctrl Pts',(0.92100307984428,1.12967372480708,-1.72169722646609));
#15211=CARTESIAN_POINT('Ctrl Pts',(0.884314808153946,0.51125562378511,-1.8890841189366));
#15212=CARTESIAN_POINT('Ctrl Pts',(0.847626536463612,-0.107162477236863,
-2.05647101140711));
#15213=CARTESIAN_POINT('Ctrl Pts',(0.810938264773279,-0.815719235606428,
-1.89092586487956));
#15214=CARTESIAN_POINT('Ctrl Pts',(0.774249993082945,-1.29582071071862,
-1.46668455020561));
#15215=CARTESIAN_POINT('Ctrl Pts',(0.742789892763374,-1.70750651314859,
-1.10289869427864));
#15216=CARTESIAN_POINT('Ctrl Pts',(0.711329792443802,-1.95120870743107,
-0.548893049517983));
#15217=CARTESIAN_POINT('Ctrl Pts',(0.67986969212423,-1.9556340392028,0.00150612460811491));
#15218=CARTESIAN_POINT('Ctrl Pts',(0.57813030787577,-1.95561149193597,0.00205040622396644));
#15219=CARTESIAN_POINT('Ctrl Pts',(0.610130081964515,-1.95125870783131,
-0.557251002244683));
#15220=CARTESIAN_POINT('Ctrl Pts',(0.642129856053259,-1.69847012498212,
-1.1214648936334));
#15221=CARTESIAN_POINT('Ctrl Pts',(0.674129630142004,-1.27449056660128,
-1.48565001922452));
#15222=CARTESIAN_POINT('Ctrl Pts',(0.710817901832338,-0.788390971463978,
-1.90319430551263));
#15223=CARTESIAN_POINT('Ctrl Pts',(0.747506173522672,-0.0772607913405855,
-2.05780072348329));
#15224=CARTESIAN_POINT('Ctrl Pts',(0.784194445213007,0.538717801437386,
-1.88129345403462));
#15225=CARTESIAN_POINT('Ctrl Pts',(0.820882716903341,1.15469639421536,-1.70478618458595));
#15226=CARTESIAN_POINT('Ctrl Pts',(0.857570988593675,1.67552339964791,-1.19716522771797));
#15227=CARTESIAN_POINT('Ctrl Pts',(0.894259260284009,1.86728135704296,-0.585977319686521));
#15228=CARTESIAN_POINT('Ctrl Pts',(0.930947531974343,2.05903931443802,0.0252105883449238));
#15229=CARTESIAN_POINT('Ctrl Pts',(0.967635803664677,1.92172822379558,0.739965447539829));
#15230=CARTESIAN_POINT('Ctrl Pts',(1.00432407535501,1.51695619911708,1.23659176882114));
#15231=CARTESIAN_POINT('Ctrl Pts',(1.04101234704534,1.11218417443858,1.73321809010245));
#15232=CARTESIAN_POINT('Ctrl Pts',(1.07770061873568,0.439951215724031,2.01171587347017));
#15233=CARTESIAN_POINT('Ctrl Pts',(1.11438889042601,-0.197448824726387,
1.94705834975702));
#15234=CARTESIAN_POINT('Ctrl Pts',(1.15107716211635,-0.834848865176806,
1.88240082604387));
#15235=CARTESIAN_POINT('Ctrl Pts',(1.18776543380668,-1.43741598736309,1.47458799524984));
#15236=CARTESIAN_POINT('Ctrl Pts',(1.22445370549701,-1.73427713098456,0.90687236394884));
#15237=CARTESIAN_POINT('Ctrl Pts',(1.24234590628993,-1.87905089503979,0.630007807497356));
#15238=CARTESIAN_POINT('Ctrl Pts',(1.26023810708285,-1.95111753748238,0.315113008990274));
#15239=CARTESIAN_POINT('Ctrl Pts',(1.27813030787577,-1.95093620579234,0.000136491009683568));
#15240=CARTESIAN_POINT('Origin',(2.1,0.,0.));
#15241=CARTESIAN_POINT('',(2.07986969212423,-1.95573740044118,-0.00134534213615312));
#15242=CARTESIAN_POINT('',(1.97813030787577,-1.95548811205351,-0.0014374884722698));
#15243=CARTESIAN_POINT('',(2.1,-1.954,-2.39295984553393E-16));
#15244=CARTESIAN_POINT('Ctrl Pts',(2.07986969212423,-1.95573740044118,-0.00134534213615312));
#15245=CARTESIAN_POINT('Ctrl Pts',(2.04823411437081,-1.9513617754685,0.552080435026859));
#15246=CARTESIAN_POINT('Ctrl Pts',(2.01659853661739,-1.70457952528747,1.10892355752443));
#15247=CARTESIAN_POINT('Ctrl Pts',(1.98496295886397,-1.28886598803054,1.47273565024201));
#15248=CARTESIAN_POINT('Ctrl Pts',(1.94827468717363,-0.806756531420955,
1.89465419416391));
#15249=CARTESIAN_POINT('Ctrl Pts',(1.9115864154833,-0.0974446001355302,
2.05695755125819));
#15250=CARTESIAN_POINT('Ctrl Pts',(1.87489814379296,0.520171110472839,1.88667626129182));
#15251=CARTESIAN_POINT('Ctrl Pts',(1.83820987210263,1.13778682108121,1.71639497132545));
#15252=CARTESIAN_POINT('Ctrl Pts',(1.8015216004123,1.66370631101252,1.21352903429844));
#15253=CARTESIAN_POINT('Ctrl Pts',(1.76483332872196,1.8614821267408,0.60416070898101));
#15254=CARTESIAN_POINT('Ctrl Pts',(1.72814505703163,2.05925794246908,-0.00520761633642043));
#15255=CARTESIAN_POINT('Ctrl Pts',(1.69145678534129,1.92889008399431,-0.721078329944262));
#15256=CARTESIAN_POINT('Ctrl Pts',(1.65476851365096,1.52899061373608,-1.22160301259317));
#15257=CARTESIAN_POINT('Ctrl Pts',(1.61808024196063,1.12909114347786,-1.72212769524207));
#15258=CARTESIAN_POINT('Ctrl Pts',(1.58139197027029,0.459660061436177,-2.00730634693204));
#15259=CARTESIAN_POINT('Ctrl Pts',(1.54470369857996,-0.178334368785628,
-1.94892793551582));
#15260=CARTESIAN_POINT('Ctrl Pts',(1.50801542688963,-0.816328799007432,
-1.89054952409961));
#15261=CARTESIAN_POINT('Ctrl Pts',(1.47132715519929,-1.42288657740936,-1.48861404957721));
#15262=CARTESIAN_POINT('Ctrl Pts',(1.43463888350896,-1.72530550827492,-0.923823214605753));
#15263=CARTESIAN_POINT('Ctrl Pts',(1.41638248638071,-1.87579174942525,-0.642778474622892));
#15264=CARTESIAN_POINT('Ctrl Pts',(1.39812608925247,-1.9509688766925,-0.321408426032222));
#15265=CARTESIAN_POINT('Ctrl Pts',(1.37986969212423,-1.95093233439697,-2.27181786092989E-5));
#15266=CARTESIAN_POINT('Ctrl Pts',(1.27813030787577,-1.95093620579234,0.000136491009683568));
#15267=CARTESIAN_POINT('Ctrl Pts',(1.29692637877319,-1.95074571367002,-0.330751868198069));
#15268=CARTESIAN_POINT('Ctrl Pts',(1.3157224496706,-1.87082328801285,-0.661730411964054));
#15269=CARTESIAN_POINT('Ctrl Pts',(1.33451852056802,-1.71170123577323,-0.948803989963511));
#15270=CARTESIAN_POINT('Ctrl Pts',(1.37120679225835,-1.40110903188379,-1.50914628076687));
#15271=CARTESIAN_POINT('Ctrl Pts',(1.40789506394869,-0.788769459048261,
-1.9022124305656));
#15272=CARTESIAN_POINT('Ctrl Pts',(1.44458333563902,-0.149992814154617,
-1.9513104881624));
#15273=CARTESIAN_POINT('Ctrl Pts',(1.48127160732935,0.488783830739032,-2.00040854575921));
#15274=CARTESIAN_POINT('Ctrl Pts',(1.51795987901969,1.15399754769079,-1.70553851115407));
#15275=CARTESIAN_POINT('Ctrl Pts',(1.55464815071002,1.54658070225749,-1.19925693841763));
#15276=CARTESIAN_POINT('Ctrl Pts',(1.59133642240036,1.93916385682417,-0.692975365681195));
#15277=CARTESIAN_POINT('Ctrl Pts',(1.62802469409069,2.0591164490058,0.0247177451865357));
#15278=CARTESIAN_POINT('Ctrl Pts',(1.66471296578102,1.85250659557346,0.631148569663603));
#15279=CARTESIAN_POINT('Ctrl Pts',(1.70140123747136,1.64589674214113,1.23757939414067));
#15280=CARTESIAN_POINT('Ctrl Pts',(1.73808950916169,1.11272444309483,1.73274793222708));
#15281=CARTESIAN_POINT('Ctrl Pts',(1.77477778085203,0.492699242176483,1.89403577002722));
#15282=CARTESIAN_POINT('Ctrl Pts',(1.81146605254236,-0.127325958741865,
2.05532360782735));
#15283=CARTESIAN_POINT('Ctrl Pts',(1.84815432423269,-0.834204061532267,
1.88273074534122));
#15284=CARTESIAN_POINT('Ctrl Pts',(1.88484259592303,-1.3101313749037,1.45385101633328));
#15285=CARTESIAN_POINT('Ctrl Pts',(1.91593849990727,-1.71351341930723,1.09034512577004));
#15286=CARTESIAN_POINT('Ctrl Pts',(1.94703440389152,-1.95098593971063,0.542728879320629));
#15287=CARTESIAN_POINT('Ctrl Pts',(1.97813030787577,-1.95548811205351,-0.0014374884722698));
#15288=CARTESIAN_POINT('Origin',(2.1,0.,0.));
#15289=CARTESIAN_POINT('',(2.77986969212423,-1.95420215314675,0.00168616502236846));
#15290=CARTESIAN_POINT('',(2.67813030787577,-1.95448068520311,0.00166033696128984));
#15291=CARTESIAN_POINT('',(2.1,-1.954,-2.39295984553393E-16));
#15292=CARTESIAN_POINT('Ctrl Pts',(2.77986969212423,-1.95420215314675,0.00168616502236846));
#15293=CARTESIAN_POINT('Ctrl Pts',(2.77171868286981,-1.95547750749154,0.144568567579198));
#15294=CARTESIAN_POINT('Ctrl Pts',(2.7635676736154,-1.94110534109393,0.287196450375289));
#15295=CARTESIAN_POINT('Ctrl Pts',(2.75541666436098,-1.91011366966327,0.426116630272658));
#15296=CARTESIAN_POINT('Ctrl Pts',(2.71872839267065,-1.77061795494924,1.05140622868445));
#15297=CARTESIAN_POINT('Ctrl Pts',(2.68204012098031,-1.29441704307028,1.60157909930793));
#15298=CARTESIAN_POINT('Ctrl Pts',(2.64535184928998,-0.695590903406722,
1.82928445128862));
#15299=CARTESIAN_POINT('Ctrl Pts',(2.60866357759965,-0.0967647637431678,
2.0569898032693));
#15300=CARTESIAN_POINT('Ctrl Pts',(2.57197530590931,0.624686603704984,1.96222763660718));
#15301=CARTESIAN_POINT('Ctrl Pts',(2.53528703421898,1.14439923861265,1.58760159088831));
#15302=CARTESIAN_POINT('Ctrl Pts',(2.49859876252864,1.66411187352032,1.21297554516944));
#15303=CARTESIAN_POINT('Ctrl Pts',(2.46191049083831,1.98208577588749,0.558485620393793));
#15304=CARTESIAN_POINT('Ctrl Pts',(2.42522221914798,1.95536747148768,-0.0816167652630086));
#15305=CARTESIAN_POINT('Ctrl Pts',(2.38853394745764,1.92864916708787,-0.721719150919808));
#15306=CARTESIAN_POINT('Ctrl Pts',(2.35184567576731,1.55723865592108,-1.34743399745777));
#15307=CARTESIAN_POINT('Ctrl Pts',(2.31515740407697,1.00811580676684,-1.67744708930463));
#15308=CARTESIAN_POINT('Ctrl Pts',(2.27846913238664,0.458992957612606,-2.0074601811515));
#15309=CARTESIAN_POINT('Ctrl Pts',(2.24178086069631,-0.267842229529066,
-2.04177151830727));
#15310=CARTESIAN_POINT('Ctrl Pts',(2.20509258900597,-0.845611821739383,
-1.76495510350447));
#15311=CARTESIAN_POINT('Ctrl Pts',(2.16840431731564,-1.4233814139497,-1.48813868870167));
#15312=CARTESIAN_POINT('Ctrl Pts',(2.1317160456253,-1.85208541122867,-0.900194521940303));
#15313=CARTESIAN_POINT('Ctrl Pts',(2.09502777393497,-1.93898391890127,-0.265455573184856));
#15314=CARTESIAN_POINT('Ctrl Pts',(2.08997507999806,-1.9509515462278,-0.178039581911978));
#15315=CARTESIAN_POINT('Ctrl Pts',(2.08492238606114,-1.95643625582299,-0.0897360486564587));
#15316=CARTESIAN_POINT('Ctrl Pts',(2.07986969212423,-1.95573740044118,-0.00134534213615312));
#15317=CARTESIAN_POINT('Ctrl Pts',(1.97813030787577,-1.95548811205351,-0.0014374884722698));
#15318=CARTESIAN_POINT('Ctrl Pts',(1.98372267558186,-1.95629779435862,-0.0993017738625638));
#15319=CARTESIAN_POINT('Ctrl Pts',(1.98931504328794,-1.94957243403652,-0.197054478603423));
#15320=CARTESIAN_POINT('Ctrl Pts',(1.99490741099403,-1.93492195755465,-0.29360461873689));
#15321=CARTESIAN_POINT('Ctrl Pts',(2.03159568268436,-1.83880870288169,-0.927013929269352));
#15322=CARTESIAN_POINT('Ctrl Pts',(2.0682839543747,-1.40160566958331,-1.50866595480452));
#15323=CARTESIAN_POINT('Ctrl Pts',(2.10497222606503,-0.819874489822593,
-1.77705709146748));
#15324=CARTESIAN_POINT('Ctrl Pts',(2.14166049775537,-0.238143310061873,
-2.04544822813044));
#15325=CARTESIAN_POINT('Ctrl Pts',(2.1783487694457,0.488116016161189,-2.00057847592119));
#15326=CARTESIAN_POINT('Ctrl Pts',(2.21503704113603,1.0323854857134,-1.66262046846173));
#15327=CARTESIAN_POINT('Ctrl Pts',(2.25172531282637,1.57665495526561,-1.32466246100228));
#15328=CARTESIAN_POINT('Ctrl Pts',(2.2884135845167,1.93893456814697,-0.693616198292611));
#15329=CARTESIAN_POINT('Ctrl Pts',(2.32510185620704,1.95634776555644,-0.0531930972874931));
#15330=CARTESIAN_POINT('Ctrl Pts',(2.36179012789737,1.97376096296591,0.587230003717631));
#15331=CARTESIAN_POINT('Ctrl Pts',(2.39847839958771,1.64630774490349,1.23702994301821));
#15332=CARTESIAN_POINT('Ctrl Pts',(2.43516667127804,1.12120682401803,1.60406418566906));
#15333=CARTESIAN_POINT('Ctrl Pts',(2.47185494296837,0.596105903132565,1.97109842831991));
#15334=CARTESIAN_POINT('Ctrl Pts',(2.50854321465871,-0.126642720575935,
2.05536697432103));
#15335=CARTESIAN_POINT('Ctrl Pts',(2.54523148634904,-0.722098404848319,
1.81898347736198));
#15336=CARTESIAN_POINT('Ctrl Pts',(2.58191975803937,-1.3175540891207,1.58259998040294));
#15337=CARTESIAN_POINT('Ctrl Pts',(2.61860802972971,-1.78571683395696,1.02556444048373));
#15338=CARTESIAN_POINT('Ctrl Pts',(2.65529630142004,-1.91610803996687,0.398313972336145));
#15339=CARTESIAN_POINT('Ctrl Pts',(2.66290763690529,-1.94315895208515,0.268184818620666));
#15340=CARTESIAN_POINT('Ctrl Pts',(2.67051897239053,-1.95567234588532,0.135033649465785));
#15341=CARTESIAN_POINT('Ctrl Pts',(2.67813030787577,-1.95448068520311,0.00166033696128984));
#15342=CARTESIAN_POINT('Origin',(2.1,0.,0.));
#15343=CARTESIAN_POINT('',(3.47986969212423,-1.95164700307266,-0.000819222043828699));
#15344=CARTESIAN_POINT('',(3.37813030787577,-1.95121195149822,-0.0006614001062776));
#15345=CARTESIAN_POINT('',(2.1,-1.954,-2.39295984553393E-16));
#15346=CARTESIAN_POINT('Ctrl Pts',(3.47986969212423,-1.95164700307266,-0.000819222043828699));
#15347=CARTESIAN_POINT('Ctrl Pts',(3.45851497967848,-1.95006730859878,0.374954087447911));
#15348=CARTESIAN_POINT('Ctrl Pts',(3.43716026723274,-1.84503254302502,0.751463634279672));
#15349=CARTESIAN_POINT('Ctrl Pts',(3.41580555478699,-1.64211448138342,1.06439633074359));
#15350=CARTESIAN_POINT('Ctrl Pts',(3.37911728309666,-1.29349293027158,1.60202753593197));
#15351=CARTESIAN_POINT('Ctrl Pts',(3.34242901140633,-0.655952689440626,
1.95200118316467));
#15352=CARTESIAN_POINT('Ctrl Pts',(3.30574073971599,-0.0154087903711613,
1.95700568946614));
#15353=CARTESIAN_POINT('Ctrl Pts',(3.26905246802566,0.625135108698308,1.96201019576761));
#15354=CARTESIAN_POINT('Ctrl Pts',(3.23236419633532,1.26868266600629,1.62204556113784));
#15355=CARTESIAN_POINT('Ctrl Pts',(3.19567592464499,1.62553032427784,1.08993855285164));
#15356=CARTESIAN_POINT('Ctrl Pts',(3.15898765295466,1.98237798254938,0.557831544565436));
#15357=CARTESIAN_POINT('Ctrl Pts',(3.12229938126432,2.0525257417845,-0.166417837377206));
#15358=CARTESIAN_POINT('Ctrl Pts',(3.08561110957399,1.80463024676985,-0.757186102430425));
#15359=CARTESIAN_POINT('Ctrl Pts',(3.04892283788365,1.55673475175519,-1.34795436748365));
#15360=CARTESIAN_POINT('Ctrl Pts',(3.01223456619332,0.99079600249076,-1.80524151564745));
#15361=CARTESIAN_POINT('Ctrl Pts',(2.97554629450299,0.361152015741564,-1.92346124918403));
#15362=CARTESIAN_POINT('Ctrl Pts',(2.93885802281265,-0.268491971007628,
-2.04168098272061));
#15363=CARTESIAN_POINT('Ctrl Pts',(2.90216975112232,-0.961841195241583,
-1.82083330162998));
#15364=CARTESIAN_POINT('Ctrl Pts',(2.86548147943198,-1.407120548584,-1.36020629798461));
#15365=CARTESIAN_POINT('Ctrl Pts',(2.83694421699607,-1.75347248009176,-1.00191649357386));
#15366=CARTESIAN_POINT('Ctrl Pts',(2.80840695456015,-1.94973704698626,-0.498555276493542));
#15367=CARTESIAN_POINT('Ctrl Pts',(2.77986969212423,-1.95420215314675,0.00168616502236846));
#15368=CARTESIAN_POINT('Ctrl Pts',(2.67813030787577,-1.95448068520311,0.00166033696128984));
#15369=CARTESIAN_POINT('Ctrl Pts',(2.70720724408086,-1.94992828546958,-0.507854360777897));
#15370=CARTESIAN_POINT('Ctrl Pts',(2.73628418028595,-1.74536376071737,-1.02061102763673));
#15371=CARTESIAN_POINT('Ctrl Pts',(2.76536111649104,-1.38719894302305,-1.38051015791529));
#15372=CARTESIAN_POINT('Ctrl Pts',(2.80204938818138,-0.935278972885786,
-1.8346184236432));
#15373=CARTESIAN_POINT('Ctrl Pts',(2.83873765987171,-0.23881936542771,-2.04536955872304));
#15374=CARTESIAN_POINT('Ctrl Pts',(2.87542593156205,0.389052003290823,-1.9180113690157));
#15375=CARTESIAN_POINT('Ctrl Pts',(2.91211420325238,1.01692337200935,-1.79065317930836));
#15376=CARTESIAN_POINT('Ctrl Pts',(2.94880247494271,1.57620650198834,-1.32518566481383));
#15377=CARTESIAN_POINT('Ctrl Pts',(2.98549074663305,1.81546846933065,-0.730879403442768));
#15378=CARTESIAN_POINT('Ctrl Pts',(3.02217901832338,2.05473043667296,-0.136573142071704));
#15379=CARTESIAN_POINT('Ctrl Pts',(3.05886729001372,1.97397124137859,0.586571866175893));
#15380=CARTESIAN_POINT('Ctrl Pts',(3.09555556170405,1.60947172480172,1.11344101728923));
#15381=CARTESIAN_POINT('Ctrl Pts',(3.13224383339438,1.24497220822485,1.64031016840256));
#15382=CARTESIAN_POINT('Ctrl Pts',(3.16893210508472,0.596732370365471,1.97090346238163));
#15383=CARTESIAN_POINT('Ctrl Pts',(3.20562037677505,-0.0437537922871413,
1.9565838232007));
#15384=CARTESIAN_POINT('Ctrl Pts',(3.24230864846539,-0.684239954939754,
1.94226418401977));
#15385=CARTESIAN_POINT('Ctrl Pts',(3.27899692015572,-1.3169724423856,1.58303161167885));
#15386=CARTESIAN_POINT('Ctrl Pts',(3.31568519184605,-1.65758271925546,1.04040462540785));
#15387=CARTESIAN_POINT('Ctrl Pts',(3.33650023052263,-1.85082747459649,0.732545977785637));
#15388=CARTESIAN_POINT('Ctrl Pts',(3.3573152691992,-1.95004264571188,0.365655528174976));
#15389=CARTESIAN_POINT('Ctrl Pts',(3.37813030787577,-1.95121195149822,-0.0006614001062776));
#15390=CARTESIAN_POINT('Origin',(-0.840056225603703,0.,0.));
#15391=CARTESIAN_POINT('',(3.7099437743963,-1.55362687475922,-0.0006521493803482));
#15392=CARTESIAN_POINT('',(3.746,-1.5555,-7.61108830709034E-15));
#15393=CARTESIAN_POINT('',(-0.840056225603703,-1.5555,-7.61108830709034E-15));
#15394=CARTESIAN_POINT('',(3.746,-1.47474487035273,-0.49467950975182));
#15395=CARTESIAN_POINT('Ctrl Pts',(3.7099437743963,-1.55362687475922,-0.000652149380348192));
#15396=CARTESIAN_POINT('Ctrl Pts',(3.7219625162642,-1.55433463120761,-0.169011276618047));
#15397=CARTESIAN_POINT('Ctrl Pts',(3.7339812581321,-1.52895516772819,-0.337184754324949));
#15398=CARTESIAN_POINT('Ctrl Pts',(3.746,-1.47669774220803,-0.496045317568146));
#15399=CARTESIAN_POINT('Origin',(3.746,0.,0.));
#15400=CARTESIAN_POINT('Origin',(-0.840056225603703,0.,0.));
#15401=CARTESIAN_POINT('',(3.0099437743963,-1.55566092590572,0.00134228745768336));
#15402=CARTESIAN_POINT('',(3.1480562256037,-1.55328054787896,-0.000526513748883434));
#15403=CARTESIAN_POINT('',(-0.840056225603703,-1.5555,-7.61108830709034E-15));
#15404=CARTESIAN_POINT('Ctrl Pts',(3.0099437743963,-1.55566092590572,0.00134228745768327));
#15405=CARTESIAN_POINT('Ctrl Pts',(3.03848103683221,-1.55210643632913,-0.396879597024407));
#15406=CARTESIAN_POINT('Ctrl Pts',(3.10370657095846,-1.19500410016139,-1.31274265575085));
#15407=CARTESIAN_POINT('Ctrl Pts',(3.20562037677505,0.33821159539077,-1.80110713232262));
#15408=CARTESIAN_POINT('Ctrl Pts',(3.31568519184605,1.6897741201822,-0.709023981398171));
#15409=CARTESIAN_POINT('Ctrl Pts',(3.42575000691706,1.52224877807848,1.02061252875298));
#15410=CARTESIAN_POINT('Ctrl Pts',(3.53581482198805,-0.0146574021557552,
1.8325086226628));
#15411=CARTESIAN_POINT('Ctrl Pts',(3.63054607781447,-1.3251033111666,1.1131477025114));
#15412=CARTESIAN_POINT('Ctrl Pts',(3.68858906195055,-1.55236934417881,0.298485712909523));
#15413=CARTESIAN_POINT('Ctrl Pts',(3.7099437743963,-1.55362687475922,-0.000652149380348192));
#15414=CARTESIAN_POINT('',(3.746,-0.947228644581641,1.23383067917929));
#15415=CARTESIAN_POINT('Origin',(3.746,0.,0.));
#15416=CARTESIAN_POINT('Ctrl Pts',(3.1480562256037,-1.55328054787896,-0.000526513748883416));
#15417=CARTESIAN_POINT('Ctrl Pts',(3.16392945861747,-1.55399038993147,-0.222903896360382));
#15418=CARTESIAN_POINT('Ctrl Pts',(3.21649096332156,-1.40604281565034,-0.958389511212442));
#15419=CARTESIAN_POINT('Ctrl Pts',(3.30574073971599,-0.283353499784069,
-1.81052838148212));
#15420=CARTESIAN_POINT('Ctrl Pts',(3.41580555478699,1.35479857128691,-1.23328473077121));
#15421=CARTESIAN_POINT('Ctrl Pts',(3.525870369858,1.77698226704399,0.452636866150692));
#15422=CARTESIAN_POINT('Ctrl Pts',(3.635935184929,0.596883679625912,1.73212294945));
#15423=CARTESIAN_POINT('Ctrl Pts',(3.70931172830967,-0.540911968892668,
1.54576553416264));
#15424=CARTESIAN_POINT('Ctrl Pts',(3.746,-0.947228644581658,1.23383067917928));
#15425=CARTESIAN_POINT('Origin',(-0.840056225603703,0.,0.));
#15426=CARTESIAN_POINT('',(2.3099437743963,-1.55688307389266,-0.00107097220715865));
#15427=CARTESIAN_POINT('',(2.4480562256037,-1.55588265395775,0.00132172678777145));
#15428=CARTESIAN_POINT('',(-0.840056225603703,-1.5555,-7.61108830709034E-15));
#15429=CARTESIAN_POINT('Ctrl Pts',(2.3099437743963,-1.55688307389266,-0.00107097220715882));
#15430=CARTESIAN_POINT('Ctrl Pts',(2.31499646833321,-1.55743940426441,-0.0714352219473509));
#15431=CARTESIAN_POINT('Ctrl Pts',(2.35673743396045,-1.52137003123898,-0.652150212445693));
#15432=CARTESIAN_POINT('Ctrl Pts',(2.43516667127804,-0.791822273096899,
-1.65268520044665));
#15433=CARTESIAN_POINT('Ctrl Pts',(2.54523148634904,0.943989600391651,-1.57074361659946));
#15434=CARTESIAN_POINT('Ctrl Pts',(2.65529630142005,1.83098404786343,-0.0764251256222896));
#15435=CARTESIAN_POINT('Ctrl Pts',(2.76536111649104,1.0716057390628,1.48661337691892));
#15436=CARTESIAN_POINT('Ctrl Pts',(2.87542593156205,-0.65134861415973,1.71292230769104));
#15437=CARTESIAN_POINT('Ctrl Pts',(2.95695348419713,-1.49373789267815,0.739678208438402));
#15438=CARTESIAN_POINT('Ctrl Pts',(3.00179276514188,-1.5566761836761,0.115085162164511));
#15439=CARTESIAN_POINT('Ctrl Pts',(3.0099437743963,-1.55566092590572,0.00134228745768327));
#15440=CARTESIAN_POINT('Ctrl Pts',(2.4480562256037,-1.55588265395775,0.0013217267877714));
#15441=CARTESIAN_POINT('Ctrl Pts',(2.4771331618088,-1.55225867351481,-0.404282220158654));
#15442=CARTESIAN_POINT('Ctrl Pts',(2.54289836970422,-1.183940345012,-1.32750035240754));
#15443=CARTESIAN_POINT('Ctrl Pts',(2.64535184928997,0.36430880065416,-1.79600600778423));
#15444=CARTESIAN_POINT('Ctrl Pts',(2.75541666436099,1.69997652125137,-0.684386685169734));
#15445=CARTESIAN_POINT('Ctrl Pts',(2.86548147943198,1.50710917998158,1.04261238391286));
#15446=CARTESIAN_POINT('Ctrl Pts',(2.97554629450299,-0.0410030018867827,
1.83212804734855));
#15447=CARTESIAN_POINT('Ctrl Pts',(3.06973787656023,-1.33415753850242,1.09794221077487));
#15448=CARTESIAN_POINT('Ctrl Pts',(3.12724118692713,-1.55234971105672,0.291083507715543));
#15449=CARTESIAN_POINT('Ctrl Pts',(3.1480562256037,-1.55328054787896,-0.000526513748883416));
#15450=CARTESIAN_POINT('Origin',(-0.840056225603703,0.,0.));
#15451=CARTESIAN_POINT('',(1.6099437743963,-1.55305795606678,-1.80850188541769E-5));
#15452=CARTESIAN_POINT('',(1.7480562256037,-1.55668462553696,-0.00114432616101223));
#15453=CARTESIAN_POINT('',(-0.840056225603703,-1.5555,-7.61108830709034E-15));
#15454=CARTESIAN_POINT('Ctrl Pts',(1.6099437743963,-1.55305795606678,-1.80850188541068E-5));
#15455=CARTESIAN_POINT('Ctrl Pts',(1.62820017152454,-1.55308704590337,-0.255860187662811));
#15456=CARTESIAN_POINT('Ctrl Pts',(1.68314484034311,-1.37297545271786,-1.02580809014116));
#15457=CARTESIAN_POINT('Ctrl Pts',(1.77477778085203,-0.166990185543427,
-1.82495415320191));
#15458=CARTESIAN_POINT('Ctrl Pts',(1.88484259592303,1.43173046151262,-1.14389674372839));
#15459=CARTESIAN_POINT('Ctrl Pts',(1.99490741099403,1.74307212557223,0.565730014230139));
#15460=CARTESIAN_POINT('Ctrl Pts',(2.10497222606503,0.487082719346801,1.76666343036964));
#15461=CARTESIAN_POINT('Ctrl Pts',(2.20998434719912,-1.12911652195273,1.39684790771125));
#15462=CARTESIAN_POINT('Ctrl Pts',(2.27830819664287,-1.55339981665366,0.439488800759608));
#15463=CARTESIAN_POINT('Ctrl Pts',(2.3099437743963,-1.55688307389266,-0.00107097220715882));
#15464=CARTESIAN_POINT('Ctrl Pts',(1.7480562256037,-1.55668462553696,-0.00114432616101215));
#15465=CARTESIAN_POINT('Ctrl Pts',(1.75364859330979,-1.55732918071895,-0.0790501070845528));
#15466=CARTESIAN_POINT('Ctrl Pts',(1.79592923270621,-1.51685231829982,-0.667378849545193));
#15467=CARTESIAN_POINT('Ctrl Pts',(1.87489814379297,-0.767721750635221,
-1.66401720492241));
#15468=CARTESIAN_POINT('Ctrl Pts',(1.98496295886397,0.966714864421041,-1.55686024551378));
#15469=CARTESIAN_POINT('Ctrl Pts',(2.09502777393497,1.83190310060879,-0.0498093832135426));
#15470=CARTESIAN_POINT('Ctrl Pts',(2.20509258900597,1.04988649769768,1.50202859874456));
#15471=CARTESIAN_POINT('Ctrl Pts',(2.31515740407697,-0.676165934510966,
1.70327689450415));
#15472=CARTESIAN_POINT('Ctrl Pts',(2.39614528294288,-1.49885377405251,0.72441565460719));
#15473=CARTESIAN_POINT('Ctrl Pts',(2.44044489011846,-1.55683128660421,0.107494801301965));
#15474=CARTESIAN_POINT('Ctrl Pts',(2.4480562256037,-1.55588265395775,0.0013217267877714));
#15475=CARTESIAN_POINT('Origin',(-0.840056225603703,0.,0.));
#15476=CARTESIAN_POINT('',(0.909943774396297,-1.55680079221082,0.00119896459975423));
#15477=CARTESIAN_POINT('',(1.0480562256037,-1.55306103792732,0.000108654946547743));
#15478=CARTESIAN_POINT('',(-0.840056225603703,-1.5555,-7.61108830709034E-15));
#15479=CARTESIAN_POINT('Ctrl Pts',(0.909943774396297,-1.55680079221082,
0.0011989645997544));
#15480=CARTESIAN_POINT('Ctrl Pts',(0.941403874715868,-1.55327796540892,
-0.436951452674117));
#15481=CARTESIAN_POINT('Ctrl Pts',(1.00955224672577,-1.13303516878223,-1.39228499895859));
#15482=CARTESIAN_POINT('Ctrl Pts',(1.11438889042601,0.478745549796269,-1.76885677260357));
#15483=CARTESIAN_POINT('Ctrl Pts',(1.22445370549702,1.74037094585896,-0.574006059349687));
#15484=CARTESIAN_POINT('Ctrl Pts',(1.33451852056802,1.4371242290595,1.13714206962872));
#15485=CARTESIAN_POINT('Ctrl Pts',(1.44458333563902,-0.158367626905839,
1.82571195327325));
#15486=CARTESIAN_POINT('Ctrl Pts',(1.53639175358178,-1.37042853583496,1.03076565848081));
#15487=CARTESIAN_POINT('Ctrl Pts',(1.5915118998342,-1.55302858662355,0.258283129098596));
#15488=CARTESIAN_POINT('Ctrl Pts',(1.6099437743963,-1.55305795606678,-1.80850188541068E-5));
#15489=CARTESIAN_POINT('Ctrl Pts',(1.0480562256037,-1.55306103792732,0.00010865494654776));
#15490=CARTESIAN_POINT('Ctrl Pts',(1.06685229650112,-1.55290939488932,-0.263298122304044));
#15491=CARTESIAN_POINT('Ctrl Pts',(1.12233663908887,-1.36509992687415,-1.04106360824864));
#15492=CARTESIAN_POINT('Ctrl Pts',(1.21450925336695,-0.140448663256852,
-1.82717801011092));
#15493=CARTESIAN_POINT('Ctrl Pts',(1.32457406843795,1.4482001648677,-1.12297585223739));
#15494=CARTESIAN_POINT('Ctrl Pts',(1.43463888350896,1.73466831809981,0.591003114939824));
#15495=CARTESIAN_POINT('Ctrl Pts',(1.54470369857996,0.461357912009977,1.77355377153154));
#15496=CARTESIAN_POINT('Ctrl Pts',(1.64917614594488,-1.14101833937308,1.38231417461337));
#15497=CARTESIAN_POINT('Ctrl Pts',(1.71696032161946,-1.55310062907875,0.432044407258565));
#15498=CARTESIAN_POINT('Ctrl Pts',(1.7480562256037,-1.55668462553696,-0.00114432616101215));
#15499=CARTESIAN_POINT('Origin',(3.746,2.59090492670967E-16,0.));
#15500=CARTESIAN_POINT('',(3.746,1.42596824066806,-1.33593808861266));
#15501=CARTESIAN_POINT('Ctrl Pts',(3.746,-1.47669774220803,-0.496045317568157));
#15502=CARTESIAN_POINT('Ctrl Pts',(3.746,-1.46767695685173,-0.541988808072643));
#15503=CARTESIAN_POINT('Ctrl Pts',(3.746,-1.45648644230582,-0.587389991070906));
#15504=CARTESIAN_POINT('Ctrl Pts',(3.746,-1.44311389873171,-0.632094361836819));
#15505=CARTESIAN_POINT('Ctrl Pts',(3.746,-1.42605782020177,-0.689112778280139));
#15506=CARTESIAN_POINT('Ctrl Pts',(3.746,-1.40545429196885,-0.744998389936387));
#15507=CARTESIAN_POINT('Ctrl Pts',(3.746,-1.38158419381388,-0.799585222171636));
#15508=CARTESIAN_POINT('Ctrl Pts',(3.746,-1.37368982492332,-0.817638293735676));
#15509=CARTESIAN_POINT('Ctrl Pts',(3.746,-1.36543774335364,-0.835549283520522));
#15510=CARTESIAN_POINT('Ctrl Pts',(3.746,-1.35683689466255,-0.853312047813334));
#15511=CARTESIAN_POINT('Ctrl Pts',(3.746,-1.35082910092434,-0.865719547110724));
#15512=CARTESIAN_POINT('Ctrl Pts',(3.746,-1.34465035509199,-0.878056205693144));
#15513=CARTESIAN_POINT('Ctrl Pts',(3.746,-1.33830595790412,-0.890315239315174));
#15514=CARTESIAN_POINT('Ctrl Pts',(3.746,-1.30979394486407,-0.945407900783096));
#15515=CARTESIAN_POINT('Ctrl Pts',(3.746,-1.27801858921512,-0.998784714934468));
#15516=CARTESIAN_POINT('Ctrl Pts',(3.746,-1.24329464671849,-1.05026739307564));
#15517=CARTESIAN_POINT('Ctrl Pts',(3.746,-1.21549197477731,-1.09148840394304));
#15518=CARTESIAN_POINT('Ctrl Pts',(3.746,-1.1857977693504,-1.13149528660234));
#15519=CARTESIAN_POINT('Ctrl Pts',(3.746,-1.15434993371631,-1.17019219952651));
#15520=CARTESIAN_POINT('Ctrl Pts',(3.746,-1.13719225263809,-1.19130491769222));
#15521=CARTESIAN_POINT('Ctrl Pts',(3.746,-1.11951222068639,-1.21202760312318));
#15522=CARTESIAN_POINT('Ctrl Pts',(3.746,-1.10132992050009,-1.23234376607124));
#15523=CARTESIAN_POINT('Ctrl Pts',(3.746,-1.09329393703457,-1.24132284725793));
#15524=CARTESIAN_POINT('Ctrl Pts',(3.746,-1.08516036012286,-1.25022177347855));
#15525=CARTESIAN_POINT('Ctrl Pts',(3.746,-1.07694000121619,-1.25902972511263));
#15526=CARTESIAN_POINT('Ctrl Pts',(3.746,-1.03283866198974,-1.30628343596823));
#15527=CARTESIAN_POINT('Ctrl Pts',(3.746,-0.986178549327218,-1.35099330214769));
#15528=CARTESIAN_POINT('Ctrl Pts',(3.746,-0.937274426077663,-1.39297381895804));
#15529=CARTESIAN_POINT('Ctrl Pts',(3.746,-0.88731744035443,-1.43585813912562));
#15530=CARTESIAN_POINT('Ctrl Pts',(3.746,-0.835018254132845,-1.47589526383444));
#15531=CARTESIAN_POINT('Ctrl Pts',(3.746,-0.780662569084495,-1.51286704790872));
#15532=CARTESIAN_POINT('Ctrl Pts',(3.746,-0.7436636018178,-1.53803309682409));
#15533=CARTESIAN_POINT('Ctrl Pts',(3.746,-0.705710755964256,-1.56177845813373));
#15534=CARTESIAN_POINT('Ctrl Pts',(3.746,-0.666883407901705,-1.58402563062414));
#15535=CARTESIAN_POINT('Ctrl Pts',(3.746,-0.645022282612557,-1.59655154983858));
#15536=CARTESIAN_POINT('Ctrl Pts',(3.746,-0.622883789925495,-1.6086023884738));
#15537=CARTESIAN_POINT('Ctrl Pts',(3.746,-0.600481117989749,-1.62016304189199));
#15538=CARTESIAN_POINT('Ctrl Pts',(3.746,-0.590196075220556,-1.62547052553442));
#15539=CARTESIAN_POINT('Ctrl Pts',(3.746,-0.579853601557955,-1.63067552933902));
#15540=CARTESIAN_POINT('Ctrl Pts',(3.746,-0.569460455658503,-1.63577381540665));
#15541=CARTESIAN_POINT('Ctrl Pts',(3.746,-0.508562938414991,-1.66564667264543));
#15542=CARTESIAN_POINT('Ctrl Pts',(3.746,-0.446154194198239,-1.69174917719426));
#15543=CARTESIAN_POINT('Ctrl Pts',(3.746,-0.382545387994772,-1.71386835327625));
#15544=CARTESIAN_POINT('Ctrl Pts',(3.746,-0.35466355323937,-1.72356391666209));
#15545=CARTESIAN_POINT('Ctrl Pts',(3.746,-0.326550579846396,-1.73249376115586));
#15546=CARTESIAN_POINT('Ctrl Pts',(3.746,-0.298230303151154,-1.74063786866498));
#15547=CARTESIAN_POINT('Ctrl Pts',(3.746,-0.235797117155308,-1.75859188035626));
#15548=CARTESIAN_POINT('Ctrl Pts',(3.746,-0.172357953747863,-1.77273055536692));
#15549=CARTESIAN_POINT('Ctrl Pts',(3.746,-0.108199968151964,-1.78319103686655));
#15550=CARTESIAN_POINT('Ctrl Pts',(3.746,-0.0745450275340682,-1.78867822416575));
#15551=CARTESIAN_POINT('Ctrl Pts',(3.746,-0.0406918803384018,-1.79315250709968));
#15552=CARTESIAN_POINT('Ctrl Pts',(3.746,-0.00667991656329378,-1.79662849654071));
#15553=CARTESIAN_POINT('Ctrl Pts',(3.746,0.0113280635103416,-1.79846889449609));
#15554=CARTESIAN_POINT('Ctrl Pts',(3.746,0.02938058296973,-1.80002938298957));
#15555=CARTESIAN_POINT('Ctrl Pts',(3.746,0.0474718931605801,-1.8013117281377));
#15556=CARTESIAN_POINT('Ctrl Pts',(3.746,0.0588526815596273,-1.80211841923035));
#15557=CARTESIAN_POINT('Ctrl Pts',(3.746,0.0702488219832869,-1.80281503367119));
#15558=CARTESIAN_POINT('Ctrl Pts',(3.746,0.0816588921433358,-1.80340195481207));
#15559=CARTESIAN_POINT('Ctrl Pts',(3.746,0.0929006830918067,-1.80398021986009));
#15560=CARTESIAN_POINT('Ctrl Pts',(3.746,0.104146803429052,-1.80445151859496));
#15561=CARTESIAN_POINT('Ctrl Pts',(3.746,0.115393905881569,-1.80481667057579));
#15562=CARTESIAN_POINT('Ctrl Pts',(3.746,0.183216213581067,-1.8070186110405));
#15563=CARTESIAN_POINT('Ctrl Pts',(3.746,0.251093954109709,-1.80536580748111));
#15564=CARTESIAN_POINT('Ctrl Pts',(3.746,0.318708653135867,-1.80002989300725));
#15565=CARTESIAN_POINT('Ctrl Pts',(3.746,0.387721529400568,-1.79458363929841));
#15566=CARTESIAN_POINT('Ctrl Pts',(3.746,0.456461268077058,-1.78530046409679));
#15567=CARTESIAN_POINT('Ctrl Pts',(3.746,0.524607649211818,-1.77231086825431));
#15568=CARTESIAN_POINT('Ctrl Pts',(3.746,0.593233643116481,-1.75922985191468));
#15569=CARTESIAN_POINT('Ctrl Pts',(3.746,0.661258933134227,-1.74239002904673));
#15570=CARTESIAN_POINT('Ctrl Pts',(3.746,0.728360259383821,-1.72187222166165));
#15571=CARTESIAN_POINT('Ctrl Pts',(3.746,0.743398135805435,-1.71727403755495));
#15572=CARTESIAN_POINT('Ctrl Pts',(3.746,0.758389586060716,-1.71249092446917));
#15573=CARTESIAN_POINT('Ctrl Pts',(3.746,0.773330913555261,-1.70752343674532));
#15574=CARTESIAN_POINT('Ctrl Pts',(3.746,0.784683538833469,-1.70374907153422));
#15575=CARTESIAN_POINT('Ctrl Pts',(3.746,0.796007432279541,-1.6998680936069));
#15576=CARTESIAN_POINT('Ctrl Pts',(3.746,0.807286588730607,-1.69588605410984));
#15577=CARTESIAN_POINT('Ctrl Pts',(3.746,0.875332946409464,-1.67186268985525));
#15578=CARTESIAN_POINT('Ctrl Pts',(3.746,0.941879691186089,-1.6441232993263));
#15579=CARTESIAN_POINT('Ctrl Pts',(3.746,1.00658917108316,-1.61281865410435));
#15580=CARTESIAN_POINT('Ctrl Pts',(3.746,1.07146563013462,-1.58143322901528));
#15581=CARTESIAN_POINT('Ctrl Pts',(3.746,1.13449641889544,-1.54646400492537));
#15582=CARTESIAN_POINT('Ctrl Pts',(3.746,1.1953402412806,-1.50801070738774));
#15583=CARTESIAN_POINT('Ctrl Pts',(3.746,1.25490827911898,-1.47036370572122));
#15584=CARTESIAN_POINT('Ctrl Pts',(3.746,1.31238108813822,-1.42937691198823));
#15585=CARTESIAN_POINT('Ctrl Pts',(3.746,1.36742213546892,-1.38509732245781));
#15586=CARTESIAN_POINT('Ctrl Pts',(3.746,1.38725915006856,-1.36913878048634));
#15587=CARTESIAN_POINT('Ctrl Pts',(3.746,1.40678007373163,-1.35275210897049));
#15588=CARTESIAN_POINT('Ctrl Pts',(3.746,1.42596824066806,-1.33593808861266));
#15589=CARTESIAN_POINT('',(3.746,-1.954,-2.39295984553393E-16));
#15590=CARTESIAN_POINT('Origin',(3.746,0.,0.));
#15591=CARTESIAN_POINT('',(3.746,1.93026759572985,0.31272288043729));
#15592=CARTESIAN_POINT('Origin',(3.746,0.,0.));
#15593=CARTESIAN_POINT('Ctrl Pts',(3.746,1.93161712722296,0.313370286892444));
#15594=CARTESIAN_POINT('Ctrl Pts',(3.746,1.9170676653561,0.369522322556259));
#15595=CARTESIAN_POINT('Ctrl Pts',(3.746,1.8998959347821,0.424871136241905));
#15596=CARTESIAN_POINT('Ctrl Pts',(3.746,1.88004233230363,0.47924162453163));
#15597=CARTESIAN_POINT('Ctrl Pts',(3.746,1.85535918428823,0.546838163325029));
#15598=CARTESIAN_POINT('Ctrl Pts',(3.746,1.82653125128417,0.612923897257949));
#15599=CARTESIAN_POINT('Ctrl Pts',(3.746,1.79383671268108,0.677242695947379));
#15600=CARTESIAN_POINT('Ctrl Pts',(3.746,1.78248277438098,0.699578893461036));
#15601=CARTESIAN_POINT('Ctrl Pts',(3.746,1.7706621870656,0.721701691516324));
#15602=CARTESIAN_POINT('Ctrl Pts',(3.746,1.75838562059073,0.743599294082916));
#15603=CARTESIAN_POINT('Ctrl Pts',(3.746,1.75113290438732,0.75653589954795));
#15604=CARTESIAN_POINT('Ctrl Pts',(3.746,1.74372103488401,0.76939389653469));
#15605=CARTESIAN_POINT('Ctrl Pts',(3.746,1.73615214576412,0.782170750034265));
#15606=CARTESIAN_POINT('Ctrl Pts',(3.746,1.72916208156856,0.79397050357335));
#15607=CARTESIAN_POINT('Ctrl Pts',(3.746,1.7220428899102,0.80569294674123));
#15608=CARTESIAN_POINT('Ctrl Pts',(3.746,1.71479708222831,0.817335825950651));
#15609=CARTESIAN_POINT('Ctrl Pts',(3.746,1.67710478427548,0.877901451131049));
#15610=CARTESIAN_POINT('Ctrl Pts',(3.746,1.63598575516677,0.93632285307313));
#15611=CARTESIAN_POINT('Ctrl Pts',(3.746,1.59171677536116,0.992351466900363));
#15612=CARTESIAN_POINT('Ctrl Pts',(3.746,1.55959936474689,1.03300056259535));
#15613=CARTESIAN_POINT('Ctrl Pts',(3.746,1.52582301942198,1.07238952467534));
#15614=CARTESIAN_POINT('Ctrl Pts',(3.746,1.49048374238826,1.11040925249883));
#15615=CARTESIAN_POINT('Ctrl Pts',(3.746,1.47779773240559,1.12405748435845));
#15616=CARTESIAN_POINT('Ctrl Pts',(3.746,1.46491025583191,1.13752914647693));
#15617=CARTESIAN_POINT('Ctrl Pts',(3.746,1.451825579104,1.15081875907035));
#15618=CARTESIAN_POINT('Ctrl Pts',(3.746,1.44285839741738,1.15992638726385));
#15619=CARTESIAN_POINT('Ctrl Pts',(3.746,1.4337969487779,1.16895011253028));
#15620=CARTESIAN_POINT('Ctrl Pts',(3.746,1.42464791636957,1.17788291675216));
#15621=CARTESIAN_POINT('Ctrl Pts',(3.746,1.37477938008039,1.22657286030263));
#15622=CARTESIAN_POINT('Ctrl Pts',(3.746,1.3224413352858,1.27243994889247));
#15623=CARTESIAN_POINT('Ctrl Pts',(3.746,1.2678925715542,1.31525763541383));
#15624=CARTESIAN_POINT('Ctrl Pts',(3.746,1.21450160441821,1.35716651725668));
#15625=CARTESIAN_POINT('Ctrl Pts',(3.746,1.15899184088837,1.39615447094));
#15626=CARTESIAN_POINT('Ctrl Pts',(3.746,1.1015848969634,1.43196503344108));
#15627=CARTESIAN_POINT('Ctrl Pts',(3.746,1.06067163266189,1.45748680673574));
#15628=CARTESIAN_POINT('Ctrl Pts',(3.746,1.01879428835795,1.48139381167139));
#15629=CARTESIAN_POINT('Ctrl Pts',(3.746,0.976030100453615,1.50357741528629));
#15630=CARTESIAN_POINT('Ctrl Pts',(3.746,0.943715750416762,1.52034024342404));
#15631=CARTESIAN_POINT('Ctrl Pts',(3.746,0.910894959489004,1.53611876003808));
#15632=CARTESIAN_POINT('Ctrl Pts',(3.746,0.877600977094349,1.55086054046809));
#15633=CARTESIAN_POINT('Ctrl Pts',(3.746,0.866501124167434,1.5557752903083));
#15634=CARTESIAN_POINT('Ctrl Pts',(3.746,0.85534698976745,1.56057547136442));
#15635=CARTESIAN_POINT('Ctrl Pts',(3.746,0.844145132007207,1.56525679972139));
#15636=CARTESIAN_POINT('Ctrl Pts',(3.746,0.783860743145455,1.59045003329939));
#15637=CARTESIAN_POINT('Ctrl Pts',(3.746,0.722418897081141,1.61211276930956));
#15638=CARTESIAN_POINT('Ctrl Pts',(3.746,0.660025508652091,1.63001714294657));
#15639=CARTESIAN_POINT('Ctrl Pts',(3.746,0.630724724982861,1.63842528028099));
#15640=CARTESIAN_POINT('Ctrl Pts',(3.746,0.601213932081696,1.64600385046251));
#15641=CARTESIAN_POINT('Ctrl Pts',(3.746,0.571513967094748,1.65272527485204));
#15642=CARTESIAN_POINT('Ctrl Pts',(3.746,0.506895215101871,1.66734919969025));
#15643=CARTESIAN_POINT('Ctrl Pts',(3.746,0.441380137523852,1.67791885103208));
#15644=CARTESIAN_POINT('Ctrl Pts',(3.746,0.375309113523308,1.68451038836656));
#15645=CARTESIAN_POINT('Ctrl Pts',(3.746,0.343701084436922,1.68766374503));
#15646=CARTESIAN_POINT('Ctrl Pts',(3.746,0.311965969078073,1.68990590810348));
#15647=CARTESIAN_POINT('Ctrl Pts',(3.746,0.280142405068005,1.69124126858452));
#15648=CARTESIAN_POINT('Ctrl Pts',(3.746,0.260904293393882,1.69204852618934));
#15649=CARTESIAN_POINT('Ctrl Pts',(3.746,0.241633879772981,1.69252434567738));
#15650=CARTESIAN_POINT('Ctrl Pts',(3.746,0.222339944596673,1.69266927819294));
#15651=CARTESIAN_POINT('Ctrl Pts',(3.746,0.211331617752912,1.69275197073269));
#15652=CARTESIAN_POINT('Ctrl Pts',(3.746,0.200313308126325,1.69272690943876));
#15653=CARTESIAN_POINT('Ctrl Pts',(3.746,0.189294283975791,1.69259425622779));
#15654=CARTESIAN_POINT('Ctrl Pts',(3.746,0.124549117359031,1.69181481749266));
#15655=CARTESIAN_POINT('Ctrl Pts',(3.746,0.0599603848989907,1.68732902375792));
#15656=CARTESIAN_POINT('Ctrl Pts',(3.746,-0.00415842200663883,1.67924353111349));
#15657=CARTESIAN_POINT('Ctrl Pts',(3.746,-0.0682057305053929,1.67116705454204));
#15658=CARTESIAN_POINT('Ctrl Pts',(3.746,-0.131785198840776,1.65949843588597));
#15659=CARTESIAN_POINT('Ctrl Pts',(3.746,-0.194566709331386,1.64429548390334));
#15660=CARTESIAN_POINT('Ctrl Pts',(3.746,-0.256180836698767,1.62937522135313));
#15661=CARTESIAN_POINT('Ctrl Pts',(3.746,-0.317027247668399,1.6110503044156));
#15662=CARTESIAN_POINT('Ctrl Pts',(3.746,-0.376763100391235,1.58933625316552));
#15663=CARTESIAN_POINT('Ctrl Pts',(3.746,-0.39261189862501,1.58357519675779));
#15664=CARTESIAN_POINT('Ctrl Pts',(3.746,-0.408382314033138,1.57757538005586));
#15665=CARTESIAN_POINT('Ctrl Pts',(3.746,-0.424067457197251,1.57133669060524));
#15666=CARTESIAN_POINT('Ctrl Pts',(3.746,-0.43438249495729,1.5672339344759));
#15667=CARTESIAN_POINT('Ctrl Pts',(3.746,-0.444660866744379,1.563027674198));
#15668=CARTESIAN_POINT('Ctrl Pts',(3.746,-0.454886794556105,1.5587239402953));
#15669=CARTESIAN_POINT('Ctrl Pts',(3.746,-0.512125342014314,1.53463424576853));
#15670=CARTESIAN_POINT('Ctrl Pts',(3.746,-0.567832044889769,1.50745156624152));
#15671=CARTESIAN_POINT('Ctrl Pts',(3.746,-0.621711649124022,1.47723387270885));
#15672=CARTESIAN_POINT('Ctrl Pts',(3.746,-0.674641683099482,1.44754873362744));
#15673=CARTESIAN_POINT('Ctrl Pts',(3.746,-0.72580917835169,1.41493409040527));
#15674=CARTESIAN_POINT('Ctrl Pts',(3.746,-0.774899315695597,1.37940945108255));
#15675=CARTESIAN_POINT('Ctrl Pts',(3.746,-0.822419019818227,1.34502127372113));
#15676=CARTESIAN_POINT('Ctrl Pts',(3.746,-0.867992618095871,1.30790580816821));
#15677=CARTESIAN_POINT('Ctrl Pts',(3.746,-0.911293112387728,1.2680547652239));
#15678=CARTESIAN_POINT('Ctrl Pts',(3.746,-0.923453836159227,1.25686280233347));
#15679=CARTESIAN_POINT('Ctrl Pts',(3.746,-0.935434990894819,1.24545493657529));
#15680=CARTESIAN_POINT('Ctrl Pts',(3.746,-0.94722864458165,1.23383067917928));
#15681=CARTESIAN_POINT('Ctrl Pts',(0.223925917727934,-0.68582572912871,
1.39614588036676));
#15682=CARTESIAN_POINT('Ctrl Pts',(0.260614189418268,-1.14559493608735,
1.17029444461958));
#15683=CARTESIAN_POINT('Ctrl Pts',(0.333990732798937,-1.81718714798608,
0.233132812382442));
#15684=CARTESIAN_POINT('Ctrl Pts',(0.444055547869938,-1.19370785634296,
-1.39197976411031));
#15685=CARTESIAN_POINT('Ctrl Pts',(0.554120362940941,0.504597663383652,
-1.76120742504176));
#15686=CARTESIAN_POINT('Ctrl Pts',(0.664185178011943,1.74842530967382,-0.548918174671008));
#15687=CARTESIAN_POINT('Ctrl Pts',(0.774249993082944,1.42050197063444,1.15804372422));
#15688=CARTESIAN_POINT('Ctrl Pts',(0.884314808153947,-0.184910056920043,
1.82314603030263));
#15689=CARTESIAN_POINT('Ctrl Pts',(0.994379623224949,-1.62394765962336,
0.849216360445764));
#15690=CARTESIAN_POINT('Ctrl Pts',(1.10444443829595,-1.60282461854704,-0.888466040798839));
#15691=CARTESIAN_POINT('Ctrl Pts',(1.21450925336695,-0.140448663256852,
-1.82717801011092));
#15692=CARTESIAN_POINT('Ctrl Pts',(1.32457406843795,1.4482001648677,-1.12297585223739));
#15693=CARTESIAN_POINT('Ctrl Pts',(1.43463888350896,1.73466831809981,0.591003114939824));
#15694=CARTESIAN_POINT('Ctrl Pts',(1.54470369857996,0.461357912009977,1.77355377153154));
#15695=CARTESIAN_POINT('Ctrl Pts',(1.65476851365096,-1.22679288976659,1.36137127777947));
#15696=CARTESIAN_POINT('Ctrl Pts',(1.76483332872196,-1.81184045835624,-0.274928577921449));
#15697=CARTESIAN_POINT('Ctrl Pts',(1.87489814379297,-0.767721750635221,
-1.66401720492241));
#15698=CARTESIAN_POINT('Ctrl Pts',(1.98496295886397,0.966714864421041,-1.55686024551378));
#15699=CARTESIAN_POINT('Ctrl Pts',(2.09502777393497,1.83190310060879,-0.0498093832135426));
#15700=CARTESIAN_POINT('Ctrl Pts',(2.20509258900597,1.04988649769768,1.50202859874456));
#15701=CARTESIAN_POINT('Ctrl Pts',(2.31515740407697,-0.676165934510966,
1.70327689450415));
#15702=CARTESIAN_POINT('Ctrl Pts',(2.42522221914797,-1.79422194719185,0.372976819256964));
#15703=CARTESIAN_POINT('Ctrl Pts',(2.53528703421898,-1.29896077877424,-1.29269476323455));
#15704=CARTESIAN_POINT('Ctrl Pts',(2.64535184928997,0.36430880065416,-1.79600600778423));
#15705=CARTESIAN_POINT('Ctrl Pts',(2.75541666436099,1.69997652125137,-0.684386685169734));
#15706=CARTESIAN_POINT('Ctrl Pts',(2.86548147943198,1.50710917998158,1.04261238391286));
#15707=CARTESIAN_POINT('Ctrl Pts',(2.97554629450299,-0.0410030018867827,
1.83212804734855));
#15708=CARTESIAN_POINT('Ctrl Pts',(3.08561110957399,-1.55208086916726,0.974216686637734));
#15709=CARTESIAN_POINT('Ctrl Pts',(3.19567592464499,-1.66787900701797,-0.75965171870431));
#15710=CARTESIAN_POINT('Ctrl Pts',(3.30574073971599,-0.283353499784069,
-1.81052838148212));
#15711=CARTESIAN_POINT('Ctrl Pts',(3.41580555478699,1.35479857128691,-1.23328473077121));
#15712=CARTESIAN_POINT('Ctrl Pts',(3.525870369858,1.77698226704399,0.452636866150692));
#15713=CARTESIAN_POINT('Ctrl Pts',(3.635935184929,0.596883679625912,1.73212294945));
#15714=CARTESIAN_POINT('Ctrl Pts',(3.70931172830967,-0.540911968892668,
1.54576553416264));
#15715=CARTESIAN_POINT('Ctrl Pts',(3.746,-0.947228644581658,1.23383067917928));
#15716=CARTESIAN_POINT('Ctrl Pts',(0.30061727848529,-0.744392439309314,
1.51537102412036));
#15717=CARTESIAN_POINT('Ctrl Pts',(0.337305550175624,-1.24342405470534,
1.27023280017104));
#15718=CARTESIAN_POINT('Ctrl Pts',(0.410682093556292,-1.97236749267106,
0.253041400346528));
#15719=CARTESIAN_POINT('Ctrl Pts',(0.520746908627293,-1.29564562142443,
-1.51084913858754));
#15720=CARTESIAN_POINT('Ctrl Pts',(0.630811723698296,0.547688238516703,
-1.91160733051249));
#15721=CARTESIAN_POINT('Ctrl Pts',(0.740876538769298,1.89773367480937,-0.595793540064002));
#15722=CARTESIAN_POINT('Ctrl Pts',(0.850941353840301,1.54180702480734,1.25693591839158));
#15723=CARTESIAN_POINT('Ctrl Pts',(0.961006168911302,-0.200700618943537,
1.97883523914771));
#15724=CARTESIAN_POINT('Ctrl Pts',(1.0710709839823,-1.76262614293203,0.921735961782452));
#15725=CARTESIAN_POINT('Ctrl Pts',(1.18113579905331,-1.73969928060447,-0.964337404188605));
#15726=CARTESIAN_POINT('Ctrl Pts',(1.29120061412431,-0.152442404242143,
-1.98321153352872));
#15727=CARTESIAN_POINT('Ctrl Pts',(1.40126542919531,1.57187053145932,-1.21887339367457));
#15728=CARTESIAN_POINT('Ctrl Pts',(1.51133024426631,1.88280189246234,0.641472361977973));
#15729=CARTESIAN_POINT('Ctrl Pts',(1.62139505933731,0.500755989356165,1.92500800445885));
#15730=CARTESIAN_POINT('Ctrl Pts',(1.73145987440832,-1.33155598128528,1.47762681280468));
#15731=CARTESIAN_POINT('Ctrl Pts',(1.84152468947932,-1.96656421763085,-0.298406353192358));
#15732=CARTESIAN_POINT('Ctrl Pts',(1.95158950455032,-0.833282045851795,
-1.80611746339484));
#15733=CARTESIAN_POINT('Ctrl Pts',(2.06165431962132,1.04926835707545,-1.6898097382465));
#15734=CARTESIAN_POINT('Ctrl Pts',(2.17171913469233,1.9883401274153,-0.054062900670009));
#15735=CARTESIAN_POINT('Ctrl Pts',(2.28178394976332,1.13954250741214,1.63029569326931));
#15736=CARTESIAN_POINT('Ctrl Pts',(2.39184876483433,-0.733907737768787,
1.84872976977681));
#15737=CARTESIAN_POINT('Ctrl Pts',(2.50191357990533,-1.94744115772564,0.40482751302615));
#15738=CARTESIAN_POINT('Ctrl Pts',(2.61197839497634,-1.40988671263078,-1.40308560501082));
#15739=CARTESIAN_POINT('Ctrl Pts',(2.72204321004733,0.395419281112895,-1.94937756979045));
#15740=CARTESIAN_POINT('Ctrl Pts',(2.83210802511834,1.84514755815669,-0.742830506886256));
#15741=CARTESIAN_POINT('Ctrl Pts',(2.94217284018934,1.63581013534913,1.13164721408307));
#15742=CARTESIAN_POINT('Ctrl Pts',(3.05223765526034,-0.0445044904224903,
1.98858428368593));
#15743=CARTESIAN_POINT('Ctrl Pts',(3.16230247033134,-1.68462222272199,1.05741080420446));
#15744=CARTESIAN_POINT('Ctrl Pts',(3.27236728540234,-1.81030904758299,-0.824522866224651));
#15745=CARTESIAN_POINT('Ctrl Pts',(3.38243210047335,-0.307550728898814,
-1.96514009476201));
#15746=CARTESIAN_POINT('Ctrl Pts',(3.49249691554435,1.47049282407976,-1.33860219894057));
#15747=CARTESIAN_POINT('Ctrl Pts',(3.60256173061535,1.92872927945522,0.491290201875763));
#15748=CARTESIAN_POINT('Ctrl Pts',(3.71262654568635,0.647855102819084,1.88003915974805));
#15749=CARTESIAN_POINT('Ctrl Pts',(3.78600308906702,-0.587103637081617,
1.67776758395666));
#15750=CARTESIAN_POINT('Ctrl Pts',(3.82269136075736,-1.02811809381894,1.33919476910812));
#15751=CARTESIAN_POINT('Ctrl Pts',(0.377308639242645,-0.802959149489918,
1.63459616787395));
#15752=CARTESIAN_POINT('Ctrl Pts',(0.413996910932979,-1.34125317332332,
1.37017115572251));
#15753=CARTESIAN_POINT('Ctrl Pts',(0.487373454313647,-2.12754783735604,
0.272949988310614));
#15754=CARTESIAN_POINT('Ctrl Pts',(0.597438269384649,-1.3975833865059,-1.62971851306476));
#15755=CARTESIAN_POINT('Ctrl Pts',(0.707503084455652,0.590778813649754,
-2.06200723598321));
#15756=CARTESIAN_POINT('Ctrl Pts',(0.817567899526653,2.04704203994491,-0.642668905456995));
#15757=CARTESIAN_POINT('Ctrl Pts',(0.927632714597656,1.66311207898024,1.35582811256316));
#15758=CARTESIAN_POINT('Ctrl Pts',(1.03769752966866,-0.216491180967031,
2.1345244479928));
#15759=CARTESIAN_POINT('Ctrl Pts',(1.14776234473966,-1.9013046262407,0.994255563119137));
#15760=CARTESIAN_POINT('Ctrl Pts',(1.25782715981066,-1.87657394266189,-1.04020876757837));
#15761=CARTESIAN_POINT('Ctrl Pts',(1.36789197488167,-0.164436145227433,
-2.13924505694653));
#15762=CARTESIAN_POINT('Ctrl Pts',(1.47795678995266,1.69554089805093,-1.31477093511175));
#15763=CARTESIAN_POINT('Ctrl Pts',(1.58802160502367,2.03093546682488,0.69194160901612));
#15764=CARTESIAN_POINT('Ctrl Pts',(1.69808642009467,0.540154066702352,2.07646223738617));
#15765=CARTESIAN_POINT('Ctrl Pts',(1.80815123516567,-1.43631907280398,1.59388234782989));
#15766=CARTESIAN_POINT('Ctrl Pts',(1.91821605023667,-2.12128797690546,-0.321884128463266));
#15767=CARTESIAN_POINT('Ctrl Pts',(2.02828086530768,-0.898842341068367,
-1.94821772186726));
#15768=CARTESIAN_POINT('Ctrl Pts',(2.13834568037868,1.13182184972985,-1.82275923097922));
#15769=CARTESIAN_POINT('Ctrl Pts',(2.24841049544968,2.14477715422182,-0.0583164181264759));
#15770=CARTESIAN_POINT('Ctrl Pts',(2.35847531052068,1.2291985171266,1.75856278779405));
#15771=CARTESIAN_POINT('Ctrl Pts',(2.46854012559169,-0.791649541026606,
1.99418264504948));
#15772=CARTESIAN_POINT('Ctrl Pts',(2.57860494066269,-2.10066036825944,0.436678206795334));
#15773=CARTESIAN_POINT('Ctrl Pts',(2.68866975573369,-1.52081264648731,-1.51347644678709));
#15774=CARTESIAN_POINT('Ctrl Pts',(2.79873457080469,0.426529761571628,-2.10274913179667));
#15775=CARTESIAN_POINT('Ctrl Pts',(2.90879938587569,1.99031859506201,-0.801274328602775));
#15776=CARTESIAN_POINT('Ctrl Pts',(3.01886420094669,1.76451109071668,1.22068204425328));
#15777=CARTESIAN_POINT('Ctrl Pts',(3.1289290160177,-0.048005978958199,2.14504052002332));
#15778=CARTESIAN_POINT('Ctrl Pts',(3.2389938310887,-1.81716357627672,1.14060492177119));
#15779=CARTESIAN_POINT('Ctrl Pts',(3.3490586461597,-1.95273908814801,-0.88939401374499));
#15780=CARTESIAN_POINT('Ctrl Pts',(3.45912346123071,-0.331747958013558,
-2.11975180804191));
#15781=CARTESIAN_POINT('Ctrl Pts',(3.5691882763017,1.58618707687261,-1.44391966710993));
#15782=CARTESIAN_POINT('Ctrl Pts',(3.67925309137271,2.08047629186646,0.529943537600835));
#15783=CARTESIAN_POINT('Ctrl Pts',(3.78931790644371,0.698826526012254,2.02795537004609));
#15784=CARTESIAN_POINT('Ctrl Pts',(3.86269444982438,-0.633295305270564,
1.80976963375068));
#15785=CARTESIAN_POINT('Ctrl Pts',(3.89938272151471,-1.10900754305623,1.44455885903696));
#15786=CARTESIAN_POINT('Ctrl Pts',(0.454,-0.861525859670522,1.75382131162755));
#15787=CARTESIAN_POINT('Ctrl Pts',(0.490688271690334,-1.4390822919413,1.47010951127397));
#15788=CARTESIAN_POINT('Ctrl Pts',(0.564064815071003,-2.28272818204102,
0.292858576274699));
#15789=CARTESIAN_POINT('Ctrl Pts',(0.674129630142004,-1.49952115158736,
-1.74858788754198));
#15790=CARTESIAN_POINT('Ctrl Pts',(0.784194445213007,0.633869388782806,
-2.21240714145394));
#15791=CARTESIAN_POINT('Ctrl Pts',(0.894259260284009,2.19635040508046,-0.689544270849986));
#15792=CARTESIAN_POINT('Ctrl Pts',(1.00432407535501,1.78441713315314,1.45472030673473));
#15793=CARTESIAN_POINT('Ctrl Pts',(1.11438889042601,-0.232281742990522,
2.29021365683789));
#15794=CARTESIAN_POINT('Ctrl Pts',(1.22445370549701,-2.03998310954937,1.06677516445582));
#15795=CARTESIAN_POINT('Ctrl Pts',(1.33451852056802,-2.01344860471932,-1.11608013096813));
#15796=CARTESIAN_POINT('Ctrl Pts',(1.44458333563902,-0.176429886212727,
-2.29527858036434));
#15797=CARTESIAN_POINT('Ctrl Pts',(1.55464815071002,1.81921126464255,-1.41066847654893));
#15798=CARTESIAN_POINT('Ctrl Pts',(1.66471296578102,2.17906904118742,0.742410856054269));
#15799=CARTESIAN_POINT('Ctrl Pts',(1.77477778085202,0.579552144048537,2.22791647031348));
#15800=CARTESIAN_POINT('Ctrl Pts',(1.88484259592303,-1.54108216432267,1.71013788285509));
#15801=CARTESIAN_POINT('Ctrl Pts',(1.99490741099403,-2.27601173618007,-0.345361903734176));
#15802=CARTESIAN_POINT('Ctrl Pts',(2.10497222606503,-0.964402636284939,
-2.09031798033969));
#15803=CARTESIAN_POINT('Ctrl Pts',(2.21503704113604,1.21437534238426,-1.95570872371194));
#15804=CARTESIAN_POINT('Ctrl Pts',(2.32510185620703,2.30121418102833,-0.0625699355829409));
#15805=CARTESIAN_POINT('Ctrl Pts',(2.43516667127804,1.31885452684106,1.88682988231879));
#15806=CARTESIAN_POINT('Ctrl Pts',(2.54523148634904,-0.849391344284427,
2.13963552032215));
#15807=CARTESIAN_POINT('Ctrl Pts',(2.65529630142005,-2.25387957879323,0.468528900564519));
#15808=CARTESIAN_POINT('Ctrl Pts',(2.76536111649104,-1.63173858034385,-1.62386728856336));
#15809=CARTESIAN_POINT('Ctrl Pts',(2.87542593156205,0.457640242030363,-2.25612069380289));
#15810=CARTESIAN_POINT('Ctrl Pts',(2.98549074663305,2.13548963196732,-0.859718150319296));
#15811=CARTESIAN_POINT('Ctrl Pts',(3.09555556170405,1.89321204608423,1.30971687442349));
#15812=CARTESIAN_POINT('Ctrl Pts',(3.20562037677505,-0.0515074674939052,
2.3014967563607));
#15813=CARTESIAN_POINT('Ctrl Pts',(3.31568519184605,-1.94970492983146,1.22379903933792));
#15814=CARTESIAN_POINT('Ctrl Pts',(3.42575000691705,-2.09516912871303,-0.95426516126533));
#15815=CARTESIAN_POINT('Ctrl Pts',(3.53581482198806,-0.355945187128305,
-2.2743635213218));
#15816=CARTESIAN_POINT('Ctrl Pts',(3.64587963705906,1.70188132966546,-1.54923713527929));
#15817=CARTESIAN_POINT('Ctrl Pts',(3.75594445213006,2.23222330427769,0.568596873325905));
#15818=CARTESIAN_POINT('Ctrl Pts',(3.86600926720106,0.749797949205426,2.17587158034414));
#15819=CARTESIAN_POINT('Ctrl Pts',(3.93938581058173,-0.679486973459512,
1.94177168354471));
#15820=CARTESIAN_POINT('Ctrl Pts',(3.97607408227207,-1.18989699229351,1.5499229489658));
#15821=CARTESIAN_POINT('Ctrl Pts',(3.37813030787577,-1.95121195149822,-0.0006614001062776));
#15822=CARTESIAN_POINT('Ctrl Pts',(3.39400354088953,-1.95210364636843,-0.280009137568746));
#15823=CARTESIAN_POINT('Ctrl Pts',(3.40987677390329,-1.89597817583308,-0.559023351935746));
#15824=CARTESIAN_POINT('Ctrl Pts',(3.42575000691705,-1.78105443863531,-0.811270854507534));
#15825=CARTESIAN_POINT('Ctrl Pts',(3.46243827860739,-1.51542781485145,-1.39429794795082));
#15826=CARTESIAN_POINT('Ctrl Pts',(3.49912655029773,-0.935686500989876,
-1.83433073463632));
#15827=CARTESIAN_POINT('Ctrl Pts',(3.53581482198806,-0.302844757926788,
-1.93349273030531));
#15828=CARTESIAN_POINT('Ctrl Pts',(3.5725030936784,0.329996985136287,-2.0326547259743));
#15829=CARTESIAN_POINT('Ctrl Pts',(3.60919136536873,1.01593915740087,-1.79094593062679));
#15830=CARTESIAN_POINT('Ctrl Pts',(3.64587963705906,1.4473005726352,-1.31711919818552));
#15831=CARTESIAN_POINT('Ctrl Pts',(3.67925309137271,1.83968810741749,-0.886103124678848));
#15832=CARTESIAN_POINT('Ctrl Pts',(3.71262654568635,2.02141985840415,-0.263018386824143));
#15833=CARTESIAN_POINT('Ctrl Pts',(3.746,1.93161712722296,0.313370286892444));
#15834=CARTESIAN_POINT('',(0.454,-0.903606778650207,-1.26612599672284));
#15835=CARTESIAN_POINT('Ctrl Pts',(0.454,-0.905483447595497,-1.26759470319303));
#15836=CARTESIAN_POINT('Ctrl Pts',(0.454,-0.946792996117872,-1.24555610748147));
#15837=CARTESIAN_POINT('Ctrl Pts',(0.454,-0.986950518103967,-1.22160057893693));
#15838=CARTESIAN_POINT('Ctrl Pts',(0.454,-1.02580464664965,-1.19576145398998));
#15839=CARTESIAN_POINT('Ctrl Pts',(0.454,-1.07536139387572,-1.16280477650245));
#15840=CARTESIAN_POINT('Ctrl Pts',(0.454,-1.12279917616985,-1.12678580943023));
#15841=CARTESIAN_POINT('Ctrl Pts',(0.453999999999999,-1.16804123571681,
-1.08802164444088));
#15842=CARTESIAN_POINT('Ctrl Pts',(0.453999999999999,-1.18300393391255,
-1.07520135050746));
#15843=CARTESIAN_POINT('Ctrl Pts',(0.454,-1.19772631758119,-1.06208038985825));
#15844=CARTESIAN_POINT('Ctrl Pts',(0.454,-1.2122051216726,-1.0486691119922));
#15845=CARTESIAN_POINT('Ctrl Pts',(0.454,-1.22231850700918,-1.03930138935026));
#15846=CARTESIAN_POINT('Ctrl Pts',(0.453999999999999,-1.23231423927351,
-1.02979084142708));
#15847=CARTESIAN_POINT('Ctrl Pts',(0.453999999999999,-1.24218737666825,
-1.02014451854826));
#15848=CARTESIAN_POINT('Ctrl Pts',(0.453999999999999,-1.28655826323154,
-0.976792959555769));
#15849=CARTESIAN_POINT('Ctrl Pts',(0.454,-1.32833546524355,-0.9308210295969));
#15850=CARTESIAN_POINT('Ctrl Pts',(0.454,-1.3674403354694,-0.882581814883813));
#15851=CARTESIAN_POINT('Ctrl Pts',(0.454,-1.39875067745407,-0.843957819943645));
#15852=CARTESIAN_POINT('Ctrl Pts',(0.454,-1.42834763673987,-0.803879070882375));
#15853=CARTESIAN_POINT('Ctrl Pts',(0.454,-1.45617979978502,-0.762505438595754));
#15854=CARTESIAN_POINT('Ctrl Pts',(0.454,-1.47136486573799,-0.73993222594365));
#15855=CARTESIAN_POINT('Ctrl Pts',(0.454,-1.48602440875415,-0.716973256869188));
#15856=CARTESIAN_POINT('Ctrl Pts',(0.454,-1.50014851923412,-0.693652552625721));
#15857=CARTESIAN_POINT('Ctrl Pts',(0.454,-1.50639086297558,-0.683345648528146));
#15858=CARTESIAN_POINT('Ctrl Pts',(0.454,-1.51252805609302,-0.672968799088347));
#15859=CARTESIAN_POINT('Ctrl Pts',(0.454,-1.51855290632997,-0.66253550249243));
#15860=CARTESIAN_POINT('Ctrl Pts',(0.454,-1.55087574256289,-0.606561706634213));
#15861=CARTESIAN_POINT('Ctrl Pts',(0.454,-1.58001862028287,-0.548883105316666));
#15862=CARTESIAN_POINT('Ctrl Pts',(0.454,-1.60589599259671,-0.489854897524755));
#15863=CARTESIAN_POINT('Ctrl Pts',(0.454,-1.63233046396166,-0.429555905429438));
#15864=CARTESIAN_POINT('Ctrl Pts',(0.454,-1.65535805931995,-0.367847793451561));
#15865=CARTESIAN_POINT('Ctrl Pts',(0.454,-1.67485353015918,-0.305067491734872));
#15866=CARTESIAN_POINT('Ctrl Pts',(0.454,-1.68812373993677,-0.262334090702869));
#15867=CARTESIAN_POINT('Ctrl Pts',(0.454,-1.69975670599144,-0.219103041221796));
#15868=CARTESIAN_POINT('Ctrl Pts',(0.454,-1.70970147254438,-0.175472883179375));
#15869=CARTESIAN_POINT('Ctrl Pts',(0.454,-1.71530078814148,-0.150907296533324));
#15870=CARTESIAN_POINT('Ctrl Pts',(0.454,-1.72036473894179,-0.12621509073321));
#15871=CARTESIAN_POINT('Ctrl Pts',(0.454,-1.72488272738576,-0.101413288871812));
#15872=CARTESIAN_POINT('Ctrl Pts',(0.454,-1.72695692636838,-0.0900268338540925));
#15873=CARTESIAN_POINT('Ctrl Pts',(0.454,-1.72891634281505,-0.0786153607655636));
#15874=CARTESIAN_POINT('Ctrl Pts',(0.454,-1.73075889574632,-0.0671865737445383));
#15875=CARTESIAN_POINT('Ctrl Pts',(0.454,-1.74155503622729,-0.000221447200933339));
#15876=CARTESIAN_POINT('Ctrl Pts',(0.454,-1.74830390754617,0.0670885593810468));
#15877=CARTESIAN_POINT('Ctrl Pts',(0.454,-1.75089263790026,0.134383670605557));
#15878=CARTESIAN_POINT('Ctrl Pts',(0.454,-1.75202734170458,0.163880763108201));
#15879=CARTESIAN_POINT('Ctrl Pts',(0.454,-1.75236223751259,0.193375422393782));
#15880=CARTESIAN_POINT('Ctrl Pts',(0.454,-1.75188513727174,0.222839010041275));
#15881=CARTESIAN_POINT('Ctrl Pts',(0.454,-1.75083332989114,0.287793953035042));
#15882=CARTESIAN_POINT('Ctrl Pts',(0.454,-1.74583870802757,0.352597407685611));
#15883=CARTESIAN_POINT('Ctrl Pts',(0.454,-1.73711625989873,0.417014750824874));
#15884=CARTESIAN_POINT('Ctrl Pts',(0.454,-1.73254078339593,0.450805727343501));
#15885=CARTESIAN_POINT('Ctrl Pts',(0.454,-1.72693866052523,0.484490621676017));
#15886=CARTESIAN_POINT('Ctrl Pts',(0.454,-1.72033536334843,0.518036023454921));
#15887=CARTESIAN_POINT('Ctrl Pts',(0.454,-1.71683918324053,0.535796963674726));
#15888=CARTESIAN_POINT('Ctrl Pts',(0.454,-1.7130622836982,0.553518800658627));
#15889=CARTESIAN_POINT('Ctrl Pts',(0.454,-1.70900803188264,0.571196551544545));
#15890=CARTESIAN_POINT('Ctrl Pts',(0.454,-1.70645760125952,0.582317192111172));
#15891=CARTESIAN_POINT('Ctrl Pts',(0.454,-1.70379740670489,0.59342038571861));
#15892=CARTESIAN_POINT('Ctrl Pts',(0.454,-1.70102823002613,0.604504883893459));
#15893=CARTESIAN_POINT('Ctrl Pts',(0.454,-1.69829989761203,0.615425890088691));
#15894=CARTESIAN_POINT('Ctrl Pts',(0.454,-1.69546799387054,0.626319814603402));
#15895=CARTESIAN_POINT('Ctrl Pts',(0.454,-1.69253427969405,0.63718369519264));
#15896=CARTESIAN_POINT('Ctrl Pts',(0.454,-1.67484336232207,0.702695194364307));
#15897=CARTESIAN_POINT('Ctrl Pts',(0.454,-1.65344939464525,0.767134543862278));
#15898=CARTESIAN_POINT('Ctrl Pts',(0.454,-1.62860949461081,0.830247232310506));
#15899=CARTESIAN_POINT('Ctrl Pts',(0.454,-1.60325594047626,0.894665002145749));
#15900=CARTESIAN_POINT('Ctrl Pts',(0.454,-1.57431228886208,0.957701558306191));
#15901=CARTESIAN_POINT('Ctrl Pts',(0.454,-1.5419968261977,1.01908871346515));
#15902=CARTESIAN_POINT('Ctrl Pts',(0.454,-1.5094539404335,1.08090788648691));
#15903=CARTESIAN_POINT('Ctrl Pts',(0.454,-1.47349128606835,1.14105534222757));
#15904=CARTESIAN_POINT('Ctrl Pts',(0.454,-1.43428052126492,1.19924548512233));
#15905=CARTESIAN_POINT('Ctrl Pts',(0.454,-1.42549303760002,1.21228641744561));
#15906=CARTESIAN_POINT('Ctrl Pts',(0.454,-1.41654222718529,1.22522896377067));
#15907=CARTESIAN_POINT('Ctrl Pts',(0.454,-1.4074296992568,1.23806975015137));
#15908=CARTESIAN_POINT('Ctrl Pts',(0.454,-1.40050600488519,1.24782617351587));
#15909=CARTESIAN_POINT('Ctrl Pts',(0.454,-1.39348872939356,1.2575239974115));
#15910=CARTESIAN_POINT('Ctrl Pts',(0.454,-1.38638785362935,1.26714953450667));
#15911=CARTESIAN_POINT('Ctrl Pts',(0.454,-1.34354833476087,1.32522031221069));
#15912=CARTESIAN_POINT('Ctrl Pts',(0.454,-1.29759234685035,1.38077208883289));
#15913=CARTESIAN_POINT('Ctrl Pts',(0.454,-1.24876265241614,1.43352592094888));
#15914=CARTESIAN_POINT('Ctrl Pts',(0.454,-1.19980697925523,1.48641585591531));
#15915=CARTESIAN_POINT('Ctrl Pts',(0.454,-1.14796231910694,1.53649439668058));
#15916=CARTESIAN_POINT('Ctrl Pts',(0.454,-1.09342367488196,1.58346421475321));
#15917=CARTESIAN_POINT('Ctrl Pts',(0.454,-1.04002865799837,1.62944911710359));
#15918=CARTESIAN_POINT('Ctrl Pts',(0.454,-0.984050882431382,1.67245516047572));
#15919=CARTESIAN_POINT('Ctrl Pts',(0.454,-0.925633527523863,1.71217418185344));
#15920=CARTESIAN_POINT('Ctrl Pts',(0.454,-0.904579654827432,1.72648909256854));
#15921=CARTESIAN_POINT('Ctrl Pts',(0.454,-0.883208561787645,1.74037670661332));
#15922=CARTESIAN_POINT('Ctrl Pts',(0.454,-0.861525859670522,1.75382131162755));
#15923=CARTESIAN_POINT('Ctrl Pts',(0.454,-0.905483447595502,-1.26759470319303));
#15924=CARTESIAN_POINT('Ctrl Pts',(0.487373454313647,-0.525928763905175,
-1.53514395112967));
#15925=CARTESIAN_POINT('Ctrl Pts',(0.557435180317628,0.542057967958432,
-1.72469696100193));
#15926=CARTESIAN_POINT('Ctrl Pts',(0.664185178011943,1.74842530967382,-0.548918174671008));
#15927=CARTESIAN_POINT('Ctrl Pts',(0.774249993082944,1.42050197063444,1.15804372422));
#15928=CARTESIAN_POINT('Ctrl Pts',(0.884314808153947,-0.184910056920043,
1.82314603030263));
#15929=CARTESIAN_POINT('Ctrl Pts',(0.975583552327533,-1.37819925413147,
1.01553700625721));
#15930=CARTESIAN_POINT('Ctrl Pts',(1.03016402481079,-1.55320538871742,0.250848661967433));
#15931=CARTESIAN_POINT('Ctrl Pts',(1.0480562256037,-1.55306103792732,0.00010865494654776));
#15932=CARTESIAN_POINT('Origin',(0.454,-2.59090492670967E-16,0.));
#15933=CARTESIAN_POINT('',(0.454000000000001,-1.954,-2.39295984553393E-16));
#15934=CARTESIAN_POINT('Origin',(0.454000000000001,0.,0.));
#15935=CARTESIAN_POINT('Origin',(0.454000000000001,0.,0.));
#15936=CARTESIAN_POINT('',(0.454,0.903606778650208,-1.26612599672284));
#15937=CARTESIAN_POINT('Ctrl Pts',(0.454,0.863551653131346,1.75602537289062));
#15938=CARTESIAN_POINT('Ctrl Pts',(0.454,0.913011386895007,1.72571903943065));
#15939=CARTESIAN_POINT('Ctrl Pts',(0.454,0.960937458194194,1.69313908228652));
#15940=CARTESIAN_POINT('Ctrl Pts',(0.454,1.00714499237834,1.65827960401643));
#15941=CARTESIAN_POINT('Ctrl Pts',(0.454,1.0645928742677,1.61494028228584));
#15942=CARTESIAN_POINT('Ctrl Pts',(0.454,1.11938591595968,1.56807765715797));
#15943=CARTESIAN_POINT('Ctrl Pts',(0.454000000000001,1.17136033785776,1.51803256103724));
#15944=CARTESIAN_POINT('Ctrl Pts',(0.454000000000001,1.18940964604431,1.50065325540726));
#15945=CARTESIAN_POINT('Ctrl Pts',(0.454,1.20711863746561,1.48288991242546));
#15946=CARTESIAN_POINT('Ctrl Pts',(0.454,1.22447914419062,1.46475618062676));
#15947=CARTESIAN_POINT('Ctrl Pts',(0.454,1.23473533695067,1.45404318406898));
#15948=CARTESIAN_POINT('Ctrl Pts',(0.454,1.24486988911837,1.44320091040706));
#15949=CARTESIAN_POINT('Ctrl Pts',(0.454,1.25488099887649,1.43223214039003));
#15950=CARTESIAN_POINT('Ctrl Pts',(0.454,1.26412654056888,1.42210217248867));
#15951=CARTESIAN_POINT('Ctrl Pts',(0.454,1.27326044703626,1.41187126626082));
#15952=CARTESIAN_POINT('Ctrl Pts',(0.454,1.28228129577652,1.40154248174902));
#15953=CARTESIAN_POINT('Ctrl Pts',(0.454,1.32920718312896,1.34781279483776));
#15954=CARTESIAN_POINT('Ctrl Pts',(0.454,1.37308198830637,1.29143148746947));
#15955=CARTESIAN_POINT('Ctrl Pts',(0.454,1.41374875944775,1.23273584565278));
#15956=CARTESIAN_POINT('Ctrl Pts',(0.454,1.44325274809575,1.19015180218825));
#15957=CARTESIAN_POINT('Ctrl Pts',(0.454,1.47106724855506,1.14634889346906));
#15958=CARTESIAN_POINT('Ctrl Pts',(0.454,1.49711593321256,1.10145078924334));
#15959=CARTESIAN_POINT('Ctrl Pts',(0.454,1.50646681252166,1.08533340138511));
#15960=CARTESIAN_POINT('Ctrl Pts',(0.454,1.51559000541425,1.06907486083694));
#15961=CARTESIAN_POINT('Ctrl Pts',(0.454,1.52448151607123,1.05268084780668));
#15962=CARTESIAN_POINT('Ctrl Pts',(0.454,1.53057504708402,1.04144570108324));
#15963=CARTESIAN_POINT('Ctrl Pts',(0.454,1.53656081317822,1.03014488360131));
#15964=CARTESIAN_POINT('Ctrl Pts',(0.454,1.54243405273428,1.01878683589326));
#15965=CARTESIAN_POINT('Ctrl Pts',(0.454,1.57444727255085,0.956877616203873));
#15966=CARTESIAN_POINT('Ctrl Pts',(0.454,1.60303973510773,0.89343041122372));
#15967=CARTESIAN_POINT('Ctrl Pts',(0.454,1.6280702961961,0.828758872414623));
#15968=CARTESIAN_POINT('Ctrl Pts',(0.454,1.6525695670393,0.765460029870219));
#15969=CARTESIAN_POINT('Ctrl Pts',(0.454,1.6736566518802,0.700987273413124));
#15970=CARTESIAN_POINT('Ctrl Pts',(0.454,1.69115094315255,0.635627431361354));
#15971=CARTESIAN_POINT('Ctrl Pts',(0.454,1.70361893851176,0.58904616695378));
#15972=CARTESIAN_POINT('Ctrl Pts',(0.454,1.71426107355774,0.542014153906118));
#15973=CARTESIAN_POINT('Ctrl Pts',(0.454,1.72299599012096,0.49463697610565));
#15974=CARTESIAN_POINT('Ctrl Pts',(0.454,1.72959643622789,0.458836919344082));
#15975=CARTESIAN_POINT('Ctrl Pts',(0.454000000000001,1.73510760988993,0.422839796026985));
#15976=CARTESIAN_POINT('Ctrl Pts',(0.454000000000001,1.73948907456737,0.386692710613922));
#15977=CARTESIAN_POINT('Ctrl Pts',(0.454000000000001,1.7409498004039,0.374641721854365));
#15978=CARTESIAN_POINT('Ctrl Pts',(0.454,1.74228510356595,0.362572258504674));
#15979=CARTESIAN_POINT('Ctrl Pts',(0.454,1.74349280108337,0.350491842553832));
#15980=CARTESIAN_POINT('Ctrl Pts',(0.454,1.74999222909259,0.285479045341838));
#15981=CARTESIAN_POINT('Ctrl Pts',(0.454,1.75277705338185,0.220389744978822));
#15982=CARTESIAN_POINT('Ctrl Pts',(0.454,1.75168943631667,0.155487404454911));
#15983=CARTESIAN_POINT('Ctrl Pts',(0.454,1.7511786721516,0.125008120127728));
#15984=CARTESIAN_POINT('Ctrl Pts',(0.454,1.74981315196432,0.0945701230721414));
#15985=CARTESIAN_POINT('Ctrl Pts',(0.454,1.74757257969712,0.0642013941078475));
#15986=CARTESIAN_POINT('Ctrl Pts',(0.454,1.74269776618386,-0.0018718553483526));
#15987=CARTESIAN_POINT('Ctrl Pts',(0.454,1.73368359948819,-0.0676189542128947));
#15988=CARTESIAN_POINT('Ctrl Pts',(0.454,1.72070227983376,-0.132736582318621));
#15989=CARTESIAN_POINT('Ctrl Pts',(0.454,1.71449208835406,-0.163888495221565));
#15990=CARTESIAN_POINT('Ctrl Pts',(0.454,1.70737328909369,-0.194895983856983));
#15991=CARTESIAN_POINT('Ctrl Pts',(0.454,1.69936136020235,-0.225723375579589));
#15992=CARTESIAN_POINT('Ctrl Pts',(0.454,1.69451799574347,-0.244359124280579));
#15993=CARTESIAN_POINT('Ctrl Pts',(0.454000000000001,1.68934820366496,-0.262929023221881));
#15994=CARTESIAN_POINT('Ctrl Pts',(0.454000000000001,1.68385507404296,-0.281424835612363));
#15995=CARTESIAN_POINT('Ctrl Pts',(0.454000000000001,1.68072088746442,-0.29197789569699));
#15996=CARTESIAN_POINT('Ctrl Pts',(0.454,1.67748072537069,-0.30250905044186));
#15997=CARTESIAN_POINT('Ctrl Pts',(0.454,1.67413744771922,-0.31300948337107));
#15998=CARTESIAN_POINT('Ctrl Pts',(0.454,1.65449317315503,-0.374707436400236));
#15999=CARTESIAN_POINT('Ctrl Pts',(0.454,1.63134961131065,-0.435173893456361));
#16000=CARTESIAN_POINT('Ctrl Pts',(0.454,1.60490028261305,-0.494140152831118));
#16001=CARTESIAN_POINT('Ctrl Pts',(0.454000000000001,1.57848042422025,-0.553040710967983));
#16002=CARTESIAN_POINT('Ctrl Pts',(0.454,1.54876141221147,-0.610445269174527));
#16003=CARTESIAN_POINT('Ctrl Pts',(0.454,1.5158949004578,-0.666054964491294));
#16004=CARTESIAN_POINT('Ctrl Pts',(0.454,1.48363949654564,-0.720630673569242));
#16005=CARTESIAN_POINT('Ctrl Pts',(0.454000000000001,1.44835179261319,-0.773478294266712));
#16006=CARTESIAN_POINT('Ctrl Pts',(0.454000000000001,1.41014670969038,-0.824274448844553));
#16007=CARTESIAN_POINT('Ctrl Pts',(0.454000000000001,1.40001039673298,-0.837751339363897));
#16008=CARTESIAN_POINT('Ctrl Pts',(0.454000000000001,1.38966860276793,-0.851083569202111));
#16009=CARTESIAN_POINT('Ctrl Pts',(0.454000000000001,1.37912323125007,-0.864264516319142));
#16010=CARTESIAN_POINT('Ctrl Pts',(0.454000000000001,1.37218815669918,-0.872932854912353));
#16011=CARTESIAN_POINT('Ctrl Pts',(0.454000000000001,1.36516478597537,-0.881535910870752));
#16012=CARTESIAN_POINT('Ctrl Pts',(0.454000000000001,1.35806349294299,-0.89006035307576));
#16013=CARTESIAN_POINT('Ctrl Pts',(0.454,1.31831518441419,-0.937774502774395));
#16014=CARTESIAN_POINT('Ctrl Pts',(0.454000000000001,1.27605572448459,-0.983120693942016));
#16015=CARTESIAN_POINT('Ctrl Pts',(0.454000000000001,1.23142674553036,-1.02583345557658));
#16016=CARTESIAN_POINT('Ctrl Pts',(0.454000000000001,1.18758428349663,-1.06779347066542));
#16017=CARTESIAN_POINT('Ctrl Pts',(0.454,1.1414543704636,-1.10721259976975));
#16018=CARTESIAN_POINT('Ctrl Pts',(0.454000000000001,1.09314756187649,-1.14379543108553));
#16019=CARTESIAN_POINT('Ctrl Pts',(0.454000000000001,1.04638611087288,-1.1792079603786));
#16020=CARTESIAN_POINT('Ctrl Pts',(0.454000000000001,0.997584202053025,
-1.2119630573062));
#16021=CARTESIAN_POINT('Ctrl Pts',(0.454000000000001,0.946829359075407,
-1.24174554702703));
#16022=CARTESIAN_POINT('Ctrl Pts',(0.454000000000001,0.932575297379321,
-1.2501097034511));
#16023=CARTESIAN_POINT('Ctrl Pts',(0.454000000000001,0.918167154629348,
-1.25823909631819));
#16024=CARTESIAN_POINT('Ctrl Pts',(0.454000000000001,0.903606778650211,
-1.26612599672283));
#16025=CARTESIAN_POINT('Origin',(0.454,0.,0.));
#16026=CARTESIAN_POINT('Origin',(-0.840056225603703,0.,0.));
#16027=CARTESIAN_POINT('Ctrl Pts',(0.454,0.903606778650207,-1.26612599672284));
#16028=CARTESIAN_POINT('Ctrl Pts',(0.490688271690334,1.32055872730335,-0.9685563961068));
#16029=CARTESIAN_POINT('Ctrl Pts',(0.564064815071002,1.83091854106863,0.0652892855698468));
#16030=CARTESIAN_POINT('Ctrl Pts',(0.674129630142005,0.951615547993874,
1.56747461872394));
#16031=CARTESIAN_POINT('Ctrl Pts',(0.784194445213006,-0.784116518650487,
1.65578585359825));
#16032=CARTESIAN_POINT('Ctrl Pts',(0.862799159964437,-1.51990443805225,
0.6571547169837));
#16033=CARTESIAN_POINT('Ctrl Pts',(0.904715603025534,-1.55738623033857,
0.0740126379323188));
#16034=CARTESIAN_POINT('Ctrl Pts',(0.909943774396297,-1.55680079221082,
0.0011989645997544));
#16035=CARTESIAN_POINT('Ctrl Pts',(0.223925917727934,1.13509973994375,-1.5904919303095));
#16036=CARTESIAN_POINT('Ctrl Pts',(0.260614189418268,1.6588696580847,-1.21668865187572));
#16037=CARTESIAN_POINT('Ctrl Pts',(0.333990732798937,2.2999773894234,0.0820155988450519));
#16038=CARTESIAN_POINT('Ctrl Pts',(0.444055547869938,1.19540776649311,1.96904236900455));
#16039=CARTESIAN_POINT('Ctrl Pts',(0.554120362940941,-0.984997542554195,
2.07997785787913));
#16040=CARTESIAN_POINT('Ctrl Pts',(0.664185178011941,-2.27921456954046,
0.323431730109015));
#16041=CARTESIAN_POINT('Ctrl Pts',(0.774249993082947,-1.52427599397599,
-1.72538071835201));
#16042=CARTESIAN_POINT('Ctrl Pts',(0.884314808153945,0.601394281132697,
-2.22201615793466));
#16043=CARTESIAN_POINT('Ctrl Pts',(0.99437962322495,2.18623261215584,-0.721059363528956));
#16044=CARTESIAN_POINT('Ctrl Pts',(1.10444443829595,1.80529781008181,1.42846390488879));
#16045=CARTESIAN_POINT('Ctrl Pts',(1.21450925336695,-0.198939468321444,
2.29343693776659));
#16046=CARTESIAN_POINT('Ctrl Pts',(1.32457406843796,-2.0242846057989,1.09626001120675));
#16047=CARTESIAN_POINT('Ctrl Pts',(1.43463888350895,-2.02944435581129,-1.08667857505481));
#16048=CARTESIAN_POINT('Ctrl Pts',(1.54470369857996,-0.209771020605504,
-2.29248499862201));
#16049=CARTESIAN_POINT('Ctrl Pts',(1.65476851365096,1.79852222551955,-1.4369490435521));
#16050=CARTESIAN_POINT('Ctrl Pts',(1.76483332872197,2.18962580094384,0.710663097271417));
#16051=CARTESIAN_POINT('Ctrl Pts',(1.87489814379296,0.61186733114989,2.21926090835247));
#16052=CARTESIAN_POINT('Ctrl Pts',(1.98496295886397,-1.51606846270638,1.73235083706963));
#16053=CARTESIAN_POINT('Ctrl Pts',(2.09502777393497,-2.28078940850763,-0.312250355178937));
#16054=CARTESIAN_POINT('Ctrl Pts',(2.20509258900597,-0.994677416670744,
-2.07608285546304));
#16055=CARTESIAN_POINT('Ctrl Pts',(2.31515740407697,1.18582814475428,-1.97314884399573));
#16056=CARTESIAN_POINT('Ctrl Pts',(2.42522221914798,2.30005967825467,-0.0960043043818408));
#16057=CARTESIAN_POINT('Ctrl Pts',(2.53528703421898,1.34613797115314,1.86746546994507));
#16058=CARTESIAN_POINT('Ctrl Pts',(2.64535184928998,-0.818216131191326,
2.15175196993141));
#16059=CARTESIAN_POINT('Ctrl Pts',(2.75541666436098,-2.24681886682819,0.501233358060979));
#16060=CARTESIAN_POINT('Ctrl Pts',(2.86548147943199,-1.65519041947554,-1.59998562053935));
#16061=CARTESIAN_POINT('Ctrl Pts',(2.97554629450299,0.424857253226333,-2.26252866381124));
#16062=CARTESIAN_POINT('Ctrl Pts',(3.08561110957399,2.12267350101962,-0.890667219319853));
#16063=CARTESIAN_POINT('Ctrl Pts',(3.19567592464499,1.91223022331427,1.28208092650808));
#16064=CARTESIAN_POINT('Ctrl Pts',(3.30574073971599,-0.0184124486096701,
2.30197483039737));
#16065=CARTESIAN_POINT('Ctrl Pts',(3.41580555478699,-1.93103317110253,1.25205388869926));
#16066=CARTESIAN_POINT('Ctrl Pts',(3.525870369858,-2.11014175528073,-0.923812400732872));
#16067=CARTESIAN_POINT('Ctrl Pts',(3.635935184929,-0.3862086545477,-2.2688026413651));
#16068=CARTESIAN_POINT('Ctrl Pts',(3.70931172830967,0.986026251664791,-1.80552819117983));
#16069=CARTESIAN_POINT('Ctrl Pts',(3.746,1.42596824066807,-1.33593808861265));
#16070=CARTESIAN_POINT('Ctrl Pts',(0.30061727848529,1.05793541951257,-1.48236995244728));
#16071=CARTESIAN_POINT('Ctrl Pts',(0.337305550175624,1.54609934782425,-1.13397789995275));
#16072=CARTESIAN_POINT('Ctrl Pts',(0.410682093556291,2.14362443997181,0.0764401610866495));
#16073=CARTESIAN_POINT('Ctrl Pts',(0.520746908627294,1.11414369366003,1.83518645224435));
#16074=CARTESIAN_POINT('Ctrl Pts',(0.630811723698295,-0.918037201252959,
1.93858052311883));
#16075=CARTESIAN_POINT('Ctrl Pts',(0.740876538769298,-2.12427308097651,
0.301444772680075));
#16076=CARTESIAN_POINT('Ctrl Pts',(0.8509413538403,-1.4206553894725,-1.60808897214537));
#16077=CARTESIAN_POINT('Ctrl Pts',(0.961006168911301,0.56051137068722,-2.07096302949096));
#16078=CARTESIAN_POINT('Ctrl Pts',(1.0710709839823,2.03761205672355,-0.672041595469201));
#16079=CARTESIAN_POINT('Ctrl Pts',(1.18113579905331,1.68257328307437,1.33135662646876));
#16080=CARTESIAN_POINT('Ctrl Pts',(1.29120061412431,-0.185415521182909,
2.13752860960214));
#16081=CARTESIAN_POINT('Ctrl Pts',(1.40126542919531,-1.88667331009592,1.02173602375095));
#16082=CARTESIAN_POINT('Ctrl Pts',(1.51133024426631,-1.89148229921102,-1.0128059356554));
#16083=CARTESIAN_POINT('Ctrl Pts',(1.62139505933732,-0.195510742251477,
-2.13664138348197));
#16084=CARTESIAN_POINT('Ctrl Pts',(1.73145987440832,1.6762583041839,-1.33926494361086));
#16085=CARTESIAN_POINT('Ctrl Pts',(1.84152468947932,2.04077457581997,0.662352069590991));
#16086=CARTESIAN_POINT('Ctrl Pts',(1.95158950455032,0.570272460548859,2.0683950823582));
#16087=CARTESIAN_POINT('Ctrl Pts',(2.06165431962132,-1.41300580791476,1.61458526071817));
#16088=CARTESIAN_POINT('Ctrl Pts',(2.17171913469233,-2.12574086205756,-0.291023509982963));
#16089=CARTESIAN_POINT('Ctrl Pts',(2.28178394976333,-0.927059035479461,
-1.93495030379091));
#16090=CARTESIAN_POINT('Ctrl Pts',(2.39184876483433,1.1052152966334,-1.83901376819698));
#16091=CARTESIAN_POINT('Ctrl Pts',(2.50191357990533,2.14370113479092,-0.0894779114619904));
#16092=CARTESIAN_POINT('Ctrl Pts',(2.61197839497633,1.25462722712303,1.74051477226969));
#16093=CARTESIAN_POINT('Ctrl Pts',(2.72204321004734,-0.762593625514126,
2.00547541585129));
#16094=CARTESIAN_POINT('Ctrl Pts',(2.83210802511834,-2.09407964498735,0.467159408353149));
#16095=CARTESIAN_POINT('Ctrl Pts',(2.94217284018934,-1.54267022463401,-1.49121825960709));
#16096=CARTESIAN_POINT('Ctrl Pts',(3.05223765526034,0.395975367281145,-2.10872148664837));
#16097=CARTESIAN_POINT('Ctrl Pts',(3.16230247033134,1.97837370740714,-0.83011947334596));
#16098=CARTESIAN_POINT('Ctrl Pts',(3.27236728540235,1.78223640823567,1.19492479392305));
#16099=CARTESIAN_POINT('Ctrl Pts',(3.38243210047334,-0.017160766458366,
2.14548609448584));
#16100=CARTESIAN_POINT('Ctrl Pts',(3.49249691554435,-1.79976112765586,1.16693900049615));
#16101=CARTESIAN_POINT('Ctrl Pts',(3.60256173061535,-1.96669387239445,-0.861011438315259));
#16102=CARTESIAN_POINT('Ctrl Pts',(3.71262654568635,-0.359954108516095,
-2.11456895788097));
#16103=CARTESIAN_POINT('Ctrl Pts',(3.78600308906702,0.918995978500612,-1.68278800281661));
#16104=CARTESIAN_POINT('Ctrl Pts',(3.82269136075736,1.32903061802968,-1.24512073475524));
#16105=CARTESIAN_POINT('Ctrl Pts',(0.377308639242645,0.980771099081388,
-1.37424797458506));
#16106=CARTESIAN_POINT('Ctrl Pts',(0.413996910932979,1.4333290375638,-1.05126714802977));
#16107=CARTESIAN_POINT('Ctrl Pts',(0.487373454313646,1.98727149052022,0.0708647233282483));
#16108=CARTESIAN_POINT('Ctrl Pts',(0.597438269384649,1.03287962082695,1.70133053548414));
#16109=CARTESIAN_POINT('Ctrl Pts',(0.707503084455651,-0.851076859951723,
1.79718318835854));
#16110=CARTESIAN_POINT('Ctrl Pts',(0.817567899526653,-1.96933159241256,
0.279457815251136));
#16111=CARTESIAN_POINT('Ctrl Pts',(0.927632714597655,-1.31703478496902,
-1.49079722593874));
#16112=CARTESIAN_POINT('Ctrl Pts',(1.03769752966866,0.519628460241746,-1.91990990104726));
#16113=CARTESIAN_POINT('Ctrl Pts',(1.14776234473966,1.88899150129125,-0.623023827409443));
#16114=CARTESIAN_POINT('Ctrl Pts',(1.25782715981066,1.55984875606694,1.23424934804874));
#16115=CARTESIAN_POINT('Ctrl Pts',(1.36789197488167,-0.171891574044375,
1.9816202814377));
#16116=CARTESIAN_POINT('Ctrl Pts',(1.47795678995266,-1.74906201439294,0.947212036295147));
#16117=CARTESIAN_POINT('Ctrl Pts',(1.58802160502367,-1.75352024261074,-0.938933296255988));
#16118=CARTESIAN_POINT('Ctrl Pts',(1.69808642009467,-0.181250463897452,
-1.98079776834194));
#16119=CARTESIAN_POINT('Ctrl Pts',(1.80815123516567,1.55399438284826,-1.24158084366963));
#16120=CARTESIAN_POINT('Ctrl Pts',(1.91821605023667,1.8919233506961,0.614041041910564));
#16121=CARTESIAN_POINT('Ctrl Pts',(2.02828086530768,0.528677589947831,1.91752925636392));
#16122=CARTESIAN_POINT('Ctrl Pts',(2.13834568037868,-1.30994315312314,1.49681968436671));
#16123=CARTESIAN_POINT('Ctrl Pts',(2.24841049544968,-1.9706923156075,-0.269796664786988));
#16124=CARTESIAN_POINT('Ctrl Pts',(2.35847531052068,-0.859440654288179,
-1.79381775211878));
#16125=CARTESIAN_POINT('Ctrl Pts',(2.46854012559169,1.02460244851252,-1.70487869239822));
#16126=CARTESIAN_POINT('Ctrl Pts',(2.57860494066268,1.98734259132718,-0.0829515185421386));
#16127=CARTESIAN_POINT('Ctrl Pts',(2.68866975573369,1.16311648309291,1.6135640745943));
#16128=CARTESIAN_POINT('Ctrl Pts',(2.79873457080469,-0.706971119836928,
1.85919886177117));
#16129=CARTESIAN_POINT('Ctrl Pts',(2.9087993858757,-1.9413404231465,0.433085458645317));
#16130=CARTESIAN_POINT('Ctrl Pts',(3.01886420094669,-1.43015002979249,-1.38245089867482));
#16131=CARTESIAN_POINT('Ctrl Pts',(3.1289290160177,0.367093481335958,-1.95491430948549));
#16132=CARTESIAN_POINT('Ctrl Pts',(3.2389938310887,1.83407391379467,-0.769571727372066));
#16133=CARTESIAN_POINT('Ctrl Pts',(3.3490586461597,1.65224259315707,1.10776866133802));
#16134=CARTESIAN_POINT('Ctrl Pts',(3.4591234612307,-0.0159090843070601,
1.98899735857432));
#16135=CARTESIAN_POINT('Ctrl Pts',(3.56918827630171,-1.6684890842092,1.08182411229303));
#16136=CARTESIAN_POINT('Ctrl Pts',(3.6792530913727,-1.82324598950817,-0.798210475897646));
#16137=CARTESIAN_POINT('Ctrl Pts',(3.78931790644371,-0.333699562484492,
-1.96033527439683));
#16138=CARTESIAN_POINT('Ctrl Pts',(3.86269444982438,0.851965705336433,-1.5600478144534));
#16139=CARTESIAN_POINT('Ctrl Pts',(3.89938272151471,1.23209299539129,-1.15430338089783));
#16140=CARTESIAN_POINT('Ctrl Pts',(0.454,0.903606778650207,-1.26612599672284));
#16141=CARTESIAN_POINT('Ctrl Pts',(0.490688271690334,1.32055872730335,-0.9685563961068));
#16142=CARTESIAN_POINT('Ctrl Pts',(0.564064815071002,1.83091854106863,0.0652892855698468));
#16143=CARTESIAN_POINT('Ctrl Pts',(0.674129630142005,0.951615547993874,
1.56747461872394));
#16144=CARTESIAN_POINT('Ctrl Pts',(0.784194445213006,-0.784116518650487,
1.65578585359825));
#16145=CARTESIAN_POINT('Ctrl Pts',(0.894259260284009,-1.81439010384861,
0.257470857822195));
#16146=CARTESIAN_POINT('Ctrl Pts',(1.00432407535501,-1.21341418046553,-1.37350547973211));
#16147=CARTESIAN_POINT('Ctrl Pts',(1.11438889042601,0.478745549796269,-1.76885677260357));
#16148=CARTESIAN_POINT('Ctrl Pts',(1.22445370549702,1.74037094585896,-0.574006059349687));
#16149=CARTESIAN_POINT('Ctrl Pts',(1.33451852056802,1.4371242290595,1.13714206962872));
#16150=CARTESIAN_POINT('Ctrl Pts',(1.44458333563902,-0.158367626905839,
1.82571195327325));
#16151=CARTESIAN_POINT('Ctrl Pts',(1.55464815071002,-1.61145071868996,0.872688048839352));
#16152=CARTESIAN_POINT('Ctrl Pts',(1.66471296578102,-1.61555818601047,-0.865060656856582));
#16153=CARTESIAN_POINT('Ctrl Pts',(1.77477778085203,-0.166990185543427,
-1.82495415320191));
#16154=CARTESIAN_POINT('Ctrl Pts',(1.88484259592303,1.43173046151262,-1.14389674372839));
#16155=CARTESIAN_POINT('Ctrl Pts',(1.99490741099403,1.74307212557223,0.565730014230139));
#16156=CARTESIAN_POINT('Ctrl Pts',(2.10497222606503,0.487082719346801,1.76666343036964));
#16157=CARTESIAN_POINT('Ctrl Pts',(2.21503704113604,-1.20688049833151,1.37905410801525));
#16158=CARTESIAN_POINT('Ctrl Pts',(2.32510185620703,-1.81564376915743,-0.248569819591012));
#16159=CARTESIAN_POINT('Ctrl Pts',(2.43516667127804,-0.791822273096899,
-1.65268520044665));
#16160=CARTESIAN_POINT('Ctrl Pts',(2.54523148634904,0.943989600391651,-1.57074361659946));
#16161=CARTESIAN_POINT('Ctrl Pts',(2.65529630142005,1.83098404786343,-0.0764251256222896));
#16162=CARTESIAN_POINT('Ctrl Pts',(2.76536111649104,1.0716057390628,1.48661337691892));
#16163=CARTESIAN_POINT('Ctrl Pts',(2.87542593156205,-0.65134861415973,1.71292230769104));
#16164=CARTESIAN_POINT('Ctrl Pts',(2.98549074663305,-1.78860120130565,0.399011508937487));
#16165=CARTESIAN_POINT('Ctrl Pts',(3.09555556170405,-1.31762983495097,-1.27368353774256));
#16166=CARTESIAN_POINT('Ctrl Pts',(3.20562037677505,0.33821159539077,-1.80110713232262));
#16167=CARTESIAN_POINT('Ctrl Pts',(3.31568519184605,1.6897741201822,-0.709023981398171));
#16168=CARTESIAN_POINT('Ctrl Pts',(3.42575000691706,1.52224877807848,1.02061252875298));
#16169=CARTESIAN_POINT('Ctrl Pts',(3.53581482198805,-0.0146574021557552,
1.8325086226628));
#16170=CARTESIAN_POINT('Ctrl Pts',(3.64587963705906,-1.53721704076253,0.996709224089919));
#16171=CARTESIAN_POINT('Ctrl Pts',(3.75594445213006,-1.67979810662189,-0.735409513480033));
#16172=CARTESIAN_POINT('Ctrl Pts',(3.86600926720107,-0.307445016452888,
-1.8061015909127));
#16173=CARTESIAN_POINT('Ctrl Pts',(3.93938581058173,0.784935432172254,-1.43730762609018));
#16174=CARTESIAN_POINT('Ctrl Pts',(3.97607408227207,1.13515537275291,-1.06348602704042));
#16175=CARTESIAN_POINT('Ctrl Pts',(3.746,1.42596824066807,-1.33593808861265));
#16176=CARTESIAN_POINT('Ctrl Pts',(3.70931172830967,0.98602625166479,-1.80552819117983));
#16177=CARTESIAN_POINT('Ctrl Pts',(3.67262345661933,0.299908798558548,-2.03716541627246));
#16178=CARTESIAN_POINT('Ctrl Pts',(3.635935184929,-0.330472111450079,-1.92881898871341));
#16179=CARTESIAN_POINT('Ctrl Pts',(3.59924691323867,-0.96085302145871,-1.82047256115436));
#16180=CARTESIAN_POINT('Ctrl Pts',(3.56255864154833,-1.53549738836972,-1.37214248094361));
#16181=CARTESIAN_POINT('Ctrl Pts',(3.525870369858,-1.79296814112886,-0.785333059266217));
#16182=CARTESIAN_POINT('Ctrl Pts',(3.51053681061341,-1.90057590947793,-0.540080922329393));
#16183=CARTESIAN_POINT('Ctrl Pts',(3.49520325136882,-1.95278128848461,-0.270639867873916));
#16184=CARTESIAN_POINT('Ctrl Pts',(3.47986969212423,-1.95164700307266,-0.000819222043828699));
#16185=CARTESIAN_POINT('Origin',(4.,1.38777878078145E-16,1.15470053837925));
#16186=CARTESIAN_POINT('',(4.,7.07050159149938E-17,1.15470053837925));
#16187=CARTESIAN_POINT('',(4.,1.,0.577350269189626));
#16188=CARTESIAN_POINT('',(4.,0.25,1.01036297108185));
#16189=CARTESIAN_POINT('',(2.,1.38777878078145E-16,1.15470053837925));
#16190=CARTESIAN_POINT('',(4.,7.07050159149938E-17,1.15470053837925));
#16191=CARTESIAN_POINT('',(2.,1.,0.577350269189626));
#16192=CARTESIAN_POINT('',(2.,1.,0.577350269189626));
#16193=CARTESIAN_POINT('',(4.,1.,0.577350269189626));
#16194=CARTESIAN_POINT('Origin',(4.,-1.,0.577350269189626));
#16195=CARTESIAN_POINT('',(4.,-1.,0.577350269189626));
#16196=CARTESIAN_POINT('',(4.,-0.75,0.721687836487032));
#16197=CARTESIAN_POINT('',(2.,-1.,0.577350269189626));
#16198=CARTESIAN_POINT('',(4.,-1.,0.577350269189626));
#16199=CARTESIAN_POINT('',(2.,7.07050159149938E-17,1.15470053837925));
#16200=CARTESIAN_POINT('Origin',(4.,-1.,-0.577350269189626));
#16201=CARTESIAN_POINT('',(4.,-1.,-0.577350269189626));
#16202=CARTESIAN_POINT('',(4.,-1.,-0.288675134594813));
#16203=CARTESIAN_POINT('',(2.,-1.,-0.577350269189626));
#16204=CARTESIAN_POINT('',(4.,-1.,-0.577350269189626));
#16205=CARTESIAN_POINT('',(2.,-1.,0.577350269189626));
#16206=CARTESIAN_POINT('Origin',(4.,-2.77555756156289E-16,-1.15470053837925));
#16207=CARTESIAN_POINT('',(4.,-2.12115047744981E-16,-1.15470053837925));
#16208=CARTESIAN_POINT('',(4.,-0.25,-1.01036297108185));
#16209=CARTESIAN_POINT('',(2.,-2.77555756156289E-16,-1.15470053837925));
#16210=CARTESIAN_POINT('',(4.,-2.12115047744981E-16,-1.15470053837925));
#16211=CARTESIAN_POINT('',(2.,-1.,-0.577350269189626));
#16212=CARTESIAN_POINT('Origin',(4.,1.,-0.577350269189626));
#16213=CARTESIAN_POINT('',(4.,1.,-0.577350269189626));
#16214=CARTESIAN_POINT('',(4.,0.75,-0.721687836487033));
#16215=CARTESIAN_POINT('',(2.,1.,-0.577350269189626));
#16216=CARTESIAN_POINT('',(4.,1.,-0.577350269189626));
#16217=CARTESIAN_POINT('',(2.,-2.12115047744981E-16,-1.15470053837925));
#16218=CARTESIAN_POINT('Origin',(4.,1.,0.577350269189626));
#16219=CARTESIAN_POINT('',(4.,1.,0.288675134594813));
#16220=CARTESIAN_POINT('',(2.,1.,-0.577350269189626));
#16221=CARTESIAN_POINT('Origin',(2.,0.,0.));
#16222=CARTESIAN_POINT('Origin',(0.,1.5,0.));
#16223=CARTESIAN_POINT('',(1.04083408558608E-16,-1.5,-1.83697019872103E-16));
#16224=CARTESIAN_POINT('Origin',(0.,0.,0.));
#16225=CARTESIAN_POINT('Origin',(0.25,0.,0.));
#16226=CARTESIAN_POINT('',(0.25,-1.75,-2.14313189850787E-16));
#16227=CARTESIAN_POINT('Origin',(2.1,0.,0.));
#16228=CARTESIAN_POINT('Origin',(3.746,0.,0.));
#16229=CARTESIAN_POINT('Origin',(3.85,0.,0.));
#16230=CARTESIAN_POINT('',(4.,-1.7,-2.0818995585505E-16));
#16231=CARTESIAN_POINT('Origin',(4.,0.,0.));
#16232=CARTESIAN_POINT('',(3.85,-1.85,-2.2655965784226E-16));
#16233=CARTESIAN_POINT('Origin',(4.,0.,0.));
#18263=UNCERTAINTY_MEASURE_WITH_UNIT(LENGTH_MEASURE(0.01),#18282,
'DISTANCE_ACCURACY_VALUE',
'Maximum model space distance between geometric entities at asserted c
onnectivities');
#18266=UNCERTAINTY_MEASURE_WITH_UNIT(LENGTH_MEASURE(0.01),#18282,
'DISTANCE_ACCURACY_VALUE',
'Maximum model space distance between geometric entities at asserted c
onnectivities');
#18278=(
GEOMETRIC_REPRESENTATION_CONTEXT(3)
GLOBAL_UNCERTAINTY_ASSIGNED_CONTEXT((#18263))
GLOBAL_UNIT_ASSIGNED_CONTEXT((#18282,#18284,#18285))
REPRESENTATION_CONTEXT('','3D')
);
#18281=(
GEOMETRIC_REPRESENTATION_CONTEXT(3)
GLOBAL_UNCERTAINTY_ASSIGNED_CONTEXT((#18266))
GLOBAL_UNIT_ASSIGNED_CONTEXT((#18282,#18284,#18285))
REPRESENTATION_CONTEXT('','3D')
);
#18282=(
LENGTH_UNIT()
NAMED_UNIT(*)
SI_UNIT(.MILLI.,.METRE.)
);
#18284=(
NAMED_UNIT(*)
PLANE_ANGLE_UNIT()
SI_UNIT($,.RADIAN.)
);
#18285=(
NAMED_UNIT(*)
SI_UNIT($,.STERADIAN.)
SOLID_ANGLE_UNIT()
);
#18297=SHAPE_DEFINITION_REPRESENTATION(#18311,#18349);
#18311=PRODUCT_DEFINITION_SHAPE('',$,#18364);
#18349=SHAPE_REPRESENTATION('',(#9847),#18278);
#18352=PRODUCT_DEFINITION_CONTEXT('part definition',#18396,'design');
#18364=PRODUCT_DEFINITION('2026-10-20-13-03-25-014',
'10_ISO_4026_Set_Screw_M4x4',#18378,#18352);
#18378=PRODUCT_DEFINITION_FORMATION('',$,#18409);
#18396=APPLICATION_CONTEXT(
'Core Data for Automotive Mechanical Design Process');
#18397=PRODUCT_CONTEXT('part definition',#18396,'mechanical');
#18409=PRODUCT('2026-10-20-13-03-25-014','10_ISO_4026_Set_Screw_M4x4',$,
(#18397));
#18475=COLOUR_RGB('Black',0.12,0.14,0.17);
#18476=FILL_AREA_STYLE_COLOUR('',#18475);
#18477=FILL_AREA_STYLE('',(#18476));
#18478=SURFACE_STYLE_FILL_AREA(#18477);
#18479=SURFACE_SIDE_STYLE('',(#18478));
#18480=SURFACE_STYLE_USAGE(.BOTH.,#18479);
#18481=PRESENTATION_STYLE_ASSIGNMENT((#18480));
ENDSEC;
END-ISO-10303-21;
